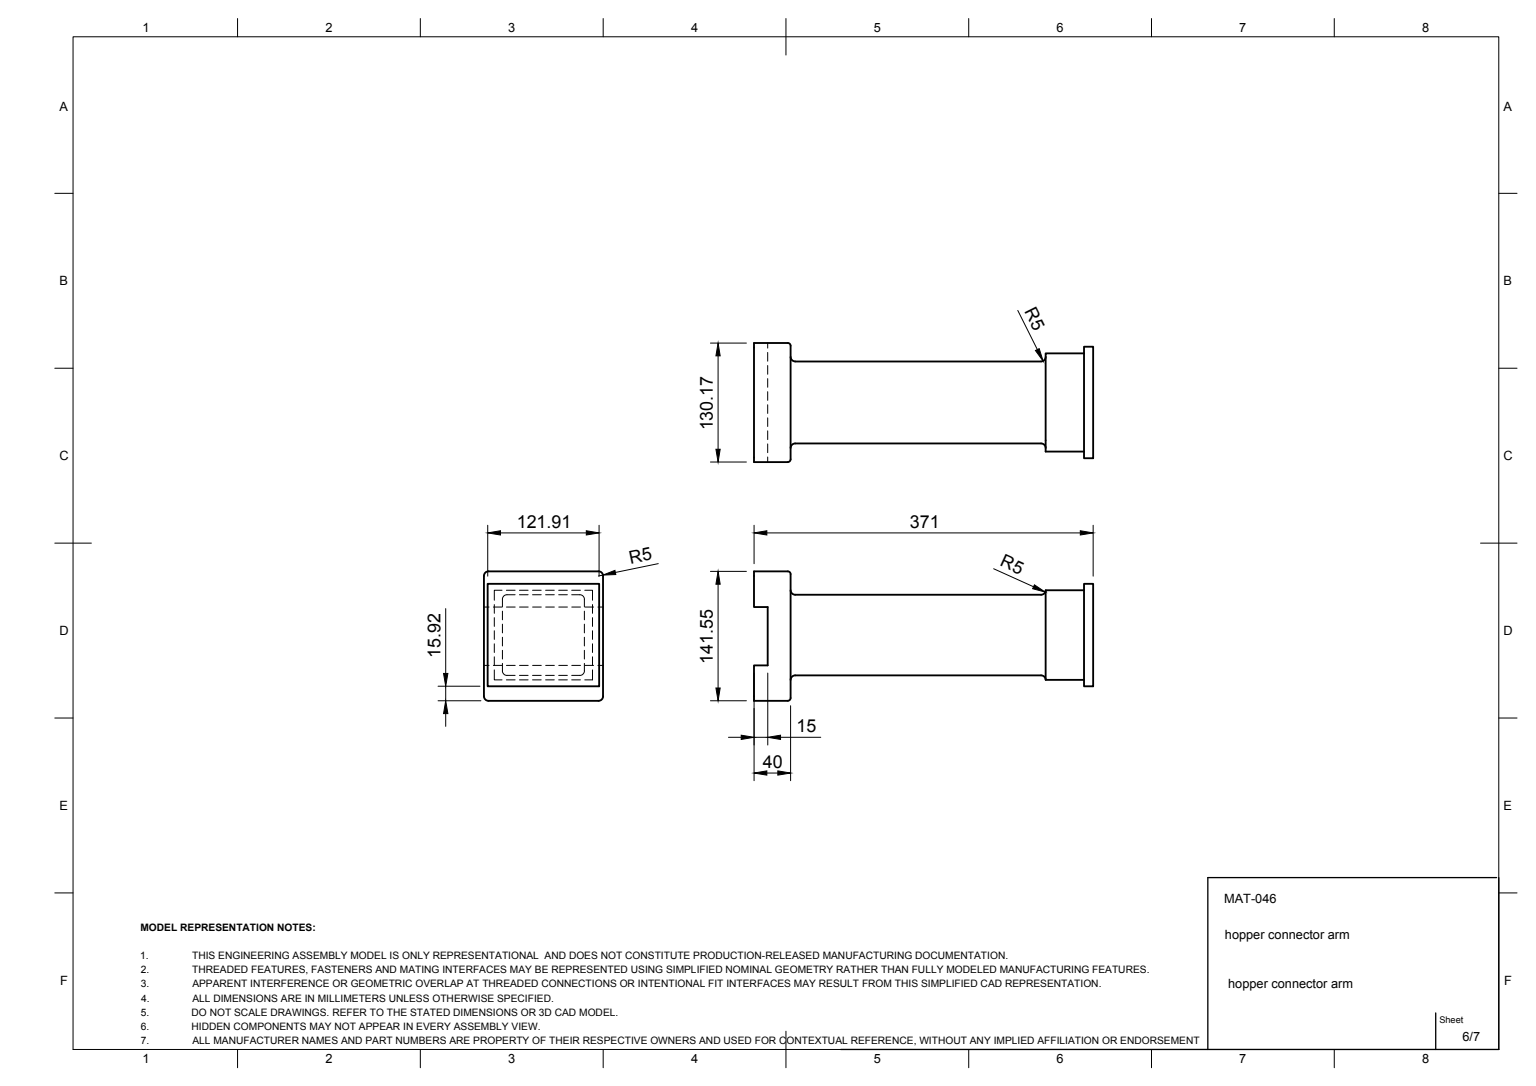
ISO-10303-21;
HEADER;
/* Generated by software containing ST-Developer
 * from STEP Tools, Inc. (www.steptools.com) 
 */

FILE_DESCRIPTION(
/* description */ ('STEP AP214'),
/* implementation_level */ '2;1');

FILE_NAME(
/* name */ 'hopper connector arm.step',
/* time_stamp */ '2026-11-14T22:16:48-08:00',
/* author */ (''),
/* organization */ (''),
/* preprocessor_version */ 'ST-DEVELOPER v20.2',
/* originating_system */ 'Autodesk Translation Framework v15.17.0.0',
/* authorisation */ '');

FILE_SCHEMA (('AUTOMOTIVE_DESIGN { 1 0 10303 214 3 1 1 }'));
ENDSEC;

DATA;
#10=MECHANICAL_DESIGN_GEOMETRIC_PRESENTATION_REPRESENTATION('',(#5499),#276462);
#4057=(
BOUNDED_SURFACE()
B_SPLINE_SURFACE(2,2,((#273891,#273892,#273893),(#273894,#273895,#273896),
(#273897,#273898,#273899)),.UNSPECIFIED.,.F.,.F.,.F.)
B_SPLINE_SURFACE_WITH_KNOTS((3,3),(3,3),(0.,1.57079632679491),(-3.14159265358979,
-1.5707963267949),.UNSPECIFIED.)
GEOMETRIC_REPRESENTATION_ITEM()
RATIONAL_B_SPLINE_SURFACE(((1.,0.707106781186548,1.),(0.707106781186546,
0.499999999999999,0.707106781186546),(1.,0.707106781186548,1.)))
REPRESENTATION_ITEM('')
SURFACE()
);
#4058=(
BOUNDED_SURFACE()
B_SPLINE_SURFACE(2,2,((#273906,#273907,#273908),(#273909,#273910,#273911),
(#273912,#273913,#273914)),.UNSPECIFIED.,.F.,.F.,.F.)
B_SPLINE_SURFACE_WITH_KNOTS((3,3),(3,3),(0.,1.57079632679491),(-1.5707963267949,
0.),.UNSPECIFIED.)
GEOMETRIC_REPRESENTATION_ITEM()
RATIONAL_B_SPLINE_SURFACE(((1.,0.707106781186547,1.),(0.707106781186542,
0.499999999999996,0.707106781186542),(1.,0.707106781186547,1.)))
REPRESENTATION_ITEM('')
SURFACE()
);
#4059=(
BOUNDED_SURFACE()
B_SPLINE_SURFACE(2,2,((#273916,#273917,#273918),(#273919,#273920,#273921),
(#273922,#273923,#273924)),.UNSPECIFIED.,.F.,.F.,.F.)
B_SPLINE_SURFACE_WITH_KNOTS((3,3),(3,3),(0.,1.57079632679491),(1.5707963267949,
3.14159265358979),.UNSPECIFIED.)
GEOMETRIC_REPRESENTATION_ITEM()
RATIONAL_B_SPLINE_SURFACE(((1.,0.707106781186548,1.),(0.707106781186542,
0.499999999999996,0.707106781186542),(1.,0.707106781186548,1.)))
REPRESENTATION_ITEM('')
SURFACE()
);
#4060=(
BOUNDED_SURFACE()
B_SPLINE_SURFACE(2,2,((#273930,#273931,#273932),(#273933,#273934,#273935),
(#273936,#273937,#273938)),.UNSPECIFIED.,.F.,.F.,.F.)
B_SPLINE_SURFACE_WITH_KNOTS((3,3),(3,3),(0.,1.57079632679491),(0.,1.5707963267949),
 .UNSPECIFIED.)
GEOMETRIC_REPRESENTATION_ITEM()
RATIONAL_B_SPLINE_SURFACE(((1.,0.707106781186548,1.),(0.707106781186542,
0.499999999999996,0.707106781186542),(1.,0.707106781186548,1.)))
REPRESENTATION_ITEM('')
SURFACE()
);
#4061=(
BOUNDED_SURFACE()
B_SPLINE_SURFACE(3,2,((#274053,#274054,#274055),(#274056,#274057,#274058),
(#274059,#274060,#274061),(#274062,#274063,#274064)),.UNSPECIFIED.,.F.,
 .F.,.F.)
B_SPLINE_SURFACE_WITH_KNOTS((4,4),(3,3),(0.00902295194197484,0.0107038053334674),
(0.,1.),.UNSPECIFIED.)
GEOMETRIC_REPRESENTATION_ITEM()
RATIONAL_B_SPLINE_SURFACE(((1.,0.717027218350901,1.),(1.,0.717027379451177,
1.),(1.,0.713716651700049,1.),(1.,0.707106781186548,1.)))
REPRESENTATION_ITEM('')
SURFACE()
);
#4062=(
BOUNDED_SURFACE()
B_SPLINE_SURFACE(3,2,((#274072,#274073,#274074),(#274075,#274076,#274077),
(#274078,#274079,#274080),(#274081,#274082,#274083)),.UNSPECIFIED.,.F.,
 .F.,.F.)
B_SPLINE_SURFACE_WITH_KNOTS((4,4),(3,3),(0.00902295194197483,0.0107038053334674),
(0.,1.),.UNSPECIFIED.)
GEOMETRIC_REPRESENTATION_ITEM()
RATIONAL_B_SPLINE_SURFACE(((1.,0.717027218350901,1.),(1.,0.717027379451176,
1.),(1.,0.713716651700055,1.),(1.,0.707106781186548,1.)))
REPRESENTATION_ITEM('')
SURFACE()
);
#4063=(
BOUNDED_SURFACE()
B_SPLINE_SURFACE(3,2,((#274085,#274086,#274087),(#274088,#274089,#274090),
(#274091,#274092,#274093),(#274094,#274095,#274096)),.UNSPECIFIED.,.F.,
 .F.,.F.)
B_SPLINE_SURFACE_WITH_KNOTS((4,4),(3,3),(0.00902295194197484,0.0107038053334674),
(0.,1.),.UNSPECIFIED.)
GEOMETRIC_REPRESENTATION_ITEM()
RATIONAL_B_SPLINE_SURFACE(((1.,0.717027218350901,1.),(1.,0.717027379451177,
1.),(1.,0.713716651700049,1.),(1.,0.707106781186548,1.)))
REPRESENTATION_ITEM('')
SURFACE()
);
#4064=(
BOUNDED_SURFACE()
B_SPLINE_SURFACE(3,2,((#274104,#274105,#274106),(#274107,#274108,#274109),
(#274110,#274111,#274112),(#274113,#274114,#274115)),.UNSPECIFIED.,.F.,
 .F.,.F.)
B_SPLINE_SURFACE_WITH_KNOTS((4,4),(3,3),(0.00902295194197484,0.0107038053334674),
(0.,1.),.UNSPECIFIED.)
GEOMETRIC_REPRESENTATION_ITEM()
RATIONAL_B_SPLINE_SURFACE(((1.,0.717027218350901,1.),(1.,0.717027379451177,
1.),(1.,0.713716651700049,1.),(1.,0.707106781186548,1.)))
REPRESENTATION_ITEM('')
SURFACE()
);
#5456=B_SPLINE_CURVE_WITH_KNOTS('',3,(#273943,#273944,#273945,#273946,#273947,
#273948,#273949,#273950,#273951,#273952),.UNSPECIFIED.,.F.,.F.,(4,3,3,4),
(0.,0.000338853006806234,0.000677883858435526,0.00084344531229996),
 .UNSPECIFIED.);
#5457=B_SPLINE_CURVE_WITH_KNOTS('',3,(#273956,#273957,#273958,#273959,#273960,
#273961,#273962,#273963,#273964,#273965),.UNSPECIFIED.,.F.,.F.,(4,3,3,4),
(0.,0.000336488810998176,0.000673156284667907,0.000840479374202616),
 .UNSPECIFIED.);
#5458=B_SPLINE_CURVE_WITH_KNOTS('',3,(#273970,#273971,#273972,#273973,#273974,
#273975,#273976,#273977,#273978,#273979),.UNSPECIFIED.,.F.,.F.,(4,3,3,4),
(0.,0.000336488811000739,0.000673156284671631,0.000840479374202609),
 .UNSPECIFIED.);
#5459=B_SPLINE_CURVE_WITH_KNOTS('',3,(#273985,#273986,#273987,#273988,#273989,
#273990,#273991,#273992,#273993,#273994),.UNSPECIFIED.,.F.,.F.,(4,3,3,4),
(0.,0.000338853006809123,0.000677883858442031,0.000843445312299953),
 .UNSPECIFIED.);
#5464=SHAPE_REPRESENTATION_RELATIONSHIP('SRR','None',#276492,#5470);
#5470=ADVANCED_BREP_SHAPE_REPRESENTATION('',(#5528),#276460);
#5499=STYLED_ITEM('',(#276527),#5528);
#5528=MANIFOLD_SOLID_BREP('Body1',#98724);
#6314=TOROIDAL_SURFACE('',#110940,10.,5.);
#6315=TOROIDAL_SURFACE('',#110947,10.,5.);
#6316=TOROIDAL_SURFACE('',#110949,10.,5.);
#6317=TOROIDAL_SURFACE('',#110955,10.,5.);
#6318=TOROIDAL_SURFACE('',#110956,10.,5.);
#6319=TOROIDAL_SURFACE('',#110964,10.,5.);
#6320=TOROIDAL_SURFACE('',#110968,10.,5.);
#6321=TOROIDAL_SURFACE('',#110975,10.,5.);
#6442=FACE_BOUND('',#19499,.T.);
#6443=FACE_BOUND('',#19546,.T.);
#7328=PLANE('',#110876);
#7329=PLANE('',#110877);
#7330=PLANE('',#110880);
#7331=PLANE('',#110881);
#7332=PLANE('',#110882);
#7333=PLANE('',#110883);
#7334=PLANE('',#110884);
#7335=PLANE('',#110893);
#7336=PLANE('',#110894);
#7337=PLANE('',#110895);
#7338=PLANE('',#110896);
#7339=PLANE('',#110933);
#7340=PLANE('',#110934);
#7341=PLANE('',#110935);
#7342=PLANE('',#110936);
#7343=PLANE('',#110937);
#7344=PLANE('',#110976);
#7345=PLANE('',#110977);
#7346=PLANE('',#110978);
#7347=PLANE('',#110979);
#7348=PLANE('',#110980);
#7349=PLANE('',#110981);
#7350=PLANE('',#110982);
#7351=PLANE('',#110983);
#7352=PLANE('',#110984);
#7353=PLANE('',#110985);
#13262=FACE_OUTER_BOUND('',#19492,.T.);
#13263=FACE_OUTER_BOUND('',#19493,.T.);
#13264=FACE_OUTER_BOUND('',#19494,.T.);
#13265=FACE_OUTER_BOUND('',#19495,.T.);
#13266=FACE_OUTER_BOUND('',#19496,.T.);
#13267=FACE_OUTER_BOUND('',#19497,.T.);
#13268=FACE_OUTER_BOUND('',#19498,.T.);
#13269=FACE_OUTER_BOUND('',#19500,.T.);
#13270=FACE_OUTER_BOUND('',#19501,.T.);
#13271=FACE_OUTER_BOUND('',#19502,.T.);
#13272=FACE_OUTER_BOUND('',#19503,.T.);
#13273=FACE_OUTER_BOUND('',#19504,.T.);
#13274=FACE_OUTER_BOUND('',#19505,.T.);
#13275=FACE_OUTER_BOUND('',#19506,.T.);
#13276=FACE_OUTER_BOUND('',#19507,.T.);
#13277=FACE_OUTER_BOUND('',#19508,.T.);
#13278=FACE_OUTER_BOUND('',#19509,.T.);
#13279=FACE_OUTER_BOUND('',#19510,.T.);
#13280=FACE_OUTER_BOUND('',#19511,.T.);
#13281=FACE_OUTER_BOUND('',#19512,.T.);
#13282=FACE_OUTER_BOUND('',#19513,.T.);
#13283=FACE_OUTER_BOUND('',#19514,.T.);
#13284=FACE_OUTER_BOUND('',#19515,.T.);
#13285=FACE_OUTER_BOUND('',#19516,.T.);
#13286=FACE_OUTER_BOUND('',#19517,.T.);
#13287=FACE_OUTER_BOUND('',#19518,.T.);
#13288=FACE_OUTER_BOUND('',#19519,.T.);
#13289=FACE_OUTER_BOUND('',#19520,.T.);
#13290=FACE_OUTER_BOUND('',#19521,.T.);
#13291=FACE_OUTER_BOUND('',#19522,.T.);
#13292=FACE_OUTER_BOUND('',#19523,.T.);
#13293=FACE_OUTER_BOUND('',#19524,.T.);
#13294=FACE_OUTER_BOUND('',#19525,.T.);
#13295=FACE_OUTER_BOUND('',#19526,.T.);
#13296=FACE_OUTER_BOUND('',#19527,.T.);
#13297=FACE_OUTER_BOUND('',#19528,.T.);
#13298=FACE_OUTER_BOUND('',#19529,.T.);
#13299=FACE_OUTER_BOUND('',#19530,.T.);
#13300=FACE_OUTER_BOUND('',#19531,.T.);
#13301=FACE_OUTER_BOUND('',#19532,.T.);
#13302=FACE_OUTER_BOUND('',#19533,.T.);
#13303=FACE_OUTER_BOUND('',#19534,.T.);
#13304=FACE_OUTER_BOUND('',#19535,.T.);
#13305=FACE_OUTER_BOUND('',#19536,.T.);
#13306=FACE_OUTER_BOUND('',#19537,.T.);
#13307=FACE_OUTER_BOUND('',#19538,.T.);
#13308=FACE_OUTER_BOUND('',#19539,.T.);
#13309=FACE_OUTER_BOUND('',#19540,.T.);
#13310=FACE_OUTER_BOUND('',#19541,.T.);
#13311=FACE_OUTER_BOUND('',#19542,.T.);
#13312=FACE_OUTER_BOUND('',#19543,.T.);
#13313=FACE_OUTER_BOUND('',#19544,.T.);
#13314=FACE_OUTER_BOUND('',#19545,.T.);
#13315=FACE_OUTER_BOUND('',#19547,.T.);
#13316=FACE_OUTER_BOUND('',#19548,.T.);
#13317=FACE_OUTER_BOUND('',#19549,.T.);
#13318=FACE_OUTER_BOUND('',#19550,.T.);
#13319=FACE_OUTER_BOUND('',#19551,.T.);
#13320=FACE_OUTER_BOUND('',#19552,.T.);
#13321=FACE_OUTER_BOUND('',#19553,.T.);
#13322=FACE_OUTER_BOUND('',#19554,.T.);
#13323=FACE_OUTER_BOUND('',#19555,.T.);
#19492=EDGE_LOOP('',(#87733,#87734,#87735,#87736));
#19493=EDGE_LOOP('',(#87737,#87738,#87739,#87740,#87741,#87742));
#19494=EDGE_LOOP('',(#87743,#87744,#87745,#87746,#87747,#87748,#87749,#87750));
#19495=EDGE_LOOP('',(#87751,#87752,#87753,#87754));
#19496=EDGE_LOOP('',(#87755,#87756,#87757,#87758,#87759,#87760,#87761,#87762));
#19497=EDGE_LOOP('',(#87763,#87764,#87765,#87766));
#19498=EDGE_LOOP('',(#87767,#87768,#87769,#87770,#87771,#87772,#87773,#87774));
#19499=EDGE_LOOP('',(#87775,#87776,#87777,#87778,#87779,#87780,#87781,#87782));
#19500=EDGE_LOOP('',(#87783,#87784,#87785,#87786));
#19501=EDGE_LOOP('',(#87787,#87788,#87789,#87790));
#19502=EDGE_LOOP('',(#87791,#87792,#87793,#87794));
#19503=EDGE_LOOP('',(#87795,#87796,#87797,#87798));
#19504=EDGE_LOOP('',(#87799,#87800,#87801,#87802));
#19505=EDGE_LOOP('',(#87803,#87804,#87805,#87806));
#19506=EDGE_LOOP('',(#87807,#87808,#87809,#87810));
#19507=EDGE_LOOP('',(#87811,#87812,#87813,#87814));
#19508=EDGE_LOOP('',(#87815,#87816,#87817,#87818));
#19509=EDGE_LOOP('',(#87819,#87820,#87821,#87822));
#19510=EDGE_LOOP('',(#87823,#87824,#87825,#87826));
#19511=EDGE_LOOP('',(#87827,#87828,#87829,#87830));
#19512=EDGE_LOOP('',(#87831,#87832,#87833,#87834));
#19513=EDGE_LOOP('',(#87835,#87836,#87837,#87838));
#19514=EDGE_LOOP('',(#87839,#87840,#87841,#87842));
#19515=EDGE_LOOP('',(#87843,#87844,#87845,#87846));
#19516=EDGE_LOOP('',(#87847,#87848,#87849,#87850,#87851));
#19517=EDGE_LOOP('',(#87852,#87853,#87854,#87855,#87856));
#19518=EDGE_LOOP('',(#87857,#87858,#87859,#87860,#87861));
#19519=EDGE_LOOP('',(#87862,#87863,#87864,#87865,#87866));
#19520=EDGE_LOOP('',(#87867,#87868,#87869,#87870));
#19521=EDGE_LOOP('',(#87871,#87872,#87873,#87874,#87875,#87876,#87877,#87878));
#19522=EDGE_LOOP('',(#87879,#87880,#87881,#87882));
#19523=EDGE_LOOP('',(#87883,#87884,#87885,#87886,#87887,#87888,#87889,#87890));
#19524=EDGE_LOOP('',(#87891,#87892,#87893,#87894,#87895,#87896));
#19525=EDGE_LOOP('',(#87897,#87898,#87899,#87900));
#19526=EDGE_LOOP('',(#87901,#87902,#87903,#87904));
#19527=EDGE_LOOP('',(#87905,#87906,#87907,#87908));
#19528=EDGE_LOOP('',(#87909,#87910,#87911,#87912));
#19529=EDGE_LOOP('',(#87913,#87914,#87915,#87916));
#19530=EDGE_LOOP('',(#87917,#87918,#87919,#87920));
#19531=EDGE_LOOP('',(#87921,#87922,#87923,#87924));
#19532=EDGE_LOOP('',(#87925,#87926,#87927,#87928));
#19533=EDGE_LOOP('',(#87929,#87930,#87931,#87932));
#19534=EDGE_LOOP('',(#87933,#87934,#87935,#87936));
#19535=EDGE_LOOP('',(#87937,#87938,#87939,#87940));
#19536=EDGE_LOOP('',(#87941,#87942,#87943,#87944));
#19537=EDGE_LOOP('',(#87945,#87946,#87947,#87948));
#19538=EDGE_LOOP('',(#87949,#87950,#87951,#87952));
#19539=EDGE_LOOP('',(#87953,#87954,#87955,#87956));
#19540=EDGE_LOOP('',(#87957,#87958,#87959,#87960));
#19541=EDGE_LOOP('',(#87961,#87962,#87963,#87964));
#19542=EDGE_LOOP('',(#87965,#87966,#87967,#87968));
#19543=EDGE_LOOP('',(#87969,#87970,#87971,#87972));
#19544=EDGE_LOOP('',(#87973,#87974,#87975,#87976));
#19545=EDGE_LOOP('',(#87977,#87978,#87979,#87980));
#19546=EDGE_LOOP('',(#87981,#87982,#87983,#87984));
#19547=EDGE_LOOP('',(#87985,#87986,#87987,#87988));
#19548=EDGE_LOOP('',(#87989,#87990,#87991,#87992));
#19549=EDGE_LOOP('',(#87993,#87994,#87995,#87996));
#19550=EDGE_LOOP('',(#87997,#87998,#87999,#88000));
#19551=EDGE_LOOP('',(#88001,#88002,#88003,#88004));
#19552=EDGE_LOOP('',(#88005,#88006,#88007,#88008));
#19553=EDGE_LOOP('',(#88009,#88010,#88011,#88012,#88013,#88014));
#19554=EDGE_LOOP('',(#88015,#88016,#88017,#88018));
#19555=EDGE_LOOP('',(#88019,#88020,#88021,#88022,#88023,#88024));
#24245=LINE('',#273745,#29472);
#24246=LINE('',#273747,#29473);
#24247=LINE('',#273749,#29474);
#24248=LINE('',#273750,#29475);
#24249=LINE('',#273754,#29476);
#24250=LINE('',#273758,#29477);
#24251=LINE('',#273760,#29478);
#24252=LINE('',#273762,#29479);
#24253=LINE('',#273767,#29480);
#24254=LINE('',#273769,#29481);
#24255=LINE('',#273771,#29482);
#24256=LINE('',#273773,#29483);
#24257=LINE('',#273774,#29484);
#24258=LINE('',#273776,#29485);
#24259=LINE('',#273777,#29486);
#24260=LINE('',#273781,#29487);
#24261=LINE('',#273783,#29488);
#24262=LINE('',#273785,#29489);
#24263=LINE('',#273786,#29490);
#24264=LINE('',#273790,#29491);
#24265=LINE('',#273792,#29492);
#24266=LINE('',#273794,#29493);
#24267=LINE('',#273796,#29494);
#24268=LINE('',#273797,#29495);
#24269=LINE('',#273799,#29496);
#24270=LINE('',#273800,#29497);
#24271=LINE('',#273804,#29498);
#24272=LINE('',#273806,#29499);
#24273=LINE('',#273808,#29500);
#24274=LINE('',#273809,#29501);
#24275=LINE('',#273813,#29502);
#24276=LINE('',#273817,#29503);
#24277=LINE('',#273821,#29504);
#24278=LINE('',#273825,#29505);
#24279=LINE('',#273829,#29506);
#24280=LINE('',#273833,#29507);
#24281=LINE('',#273837,#29508);
#24282=LINE('',#273841,#29509);
#24283=LINE('',#273846,#29510);
#24284=LINE('',#273848,#29511);
#24285=LINE('',#273850,#29512);
#24286=LINE('',#273851,#29513);
#24287=LINE('',#273855,#29514);
#24288=LINE('',#273857,#29515);
#24289=LINE('',#273859,#29516);
#24290=LINE('',#273860,#29517);
#24291=LINE('',#273864,#29518);
#24292=LINE('',#273866,#29519);
#24293=LINE('',#273868,#29520);
#24294=LINE('',#273869,#29521);
#24295=LINE('',#273873,#29522);
#24296=LINE('',#273875,#29523);
#24297=LINE('',#273877,#29524);
#24298=LINE('',#273878,#29525);
#24299=LINE('',#273997,#29526);
#24300=LINE('',#273999,#29527);
#24301=LINE('',#274000,#29528);
#24302=LINE('',#274003,#29529);
#24303=LINE('',#274005,#29530);
#24304=LINE('',#274007,#29531);
#24305=LINE('',#274009,#29532);
#24306=LINE('',#274011,#29533);
#24307=LINE('',#274012,#29534);
#24308=LINE('',#274015,#29535);
#24309=LINE('',#274017,#29536);
#24310=LINE('',#274018,#29537);
#24311=LINE('',#274021,#29538);
#24312=LINE('',#274023,#29539);
#24313=LINE('',#274025,#29540);
#24314=LINE('',#274026,#29541);
#24315=LINE('',#274027,#29542);
#24316=LINE('',#274031,#29543);
#24317=LINE('',#274121,#29544);
#24318=LINE('',#274123,#29545);
#24319=LINE('',#274125,#29546);
#24320=LINE('',#274126,#29547);
#24321=LINE('',#274129,#29548);
#24322=LINE('',#274131,#29549);
#24323=LINE('',#274132,#29550);
#24324=LINE('',#274135,#29551);
#24325=LINE('',#274136,#29552);
#24326=LINE('',#274139,#29553);
#24327=LINE('',#274140,#29554);
#24328=LINE('',#274142,#29555);
#24329=LINE('',#274145,#29556);
#24330=LINE('',#274148,#29557);
#29472=VECTOR('',#140110,1000.);
#29473=VECTOR('',#140111,1000.);
#29474=VECTOR('',#140112,1000.);
#29475=VECTOR('',#140113,1000.);
#29476=VECTOR('',#140116,1000.);
#29477=VECTOR('',#140119,1000.);
#29478=VECTOR('',#140120,1000.);
#29479=VECTOR('',#140121,1000.);
#29480=VECTOR('',#140126,1000.);
#29481=VECTOR('',#140127,1000.);
#29482=VECTOR('',#140128,1000.);
#29483=VECTOR('',#140129,1000.);
#29484=VECTOR('',#140130,1000.);
#29485=VECTOR('',#140131,1000.);
#29486=VECTOR('',#140132,1000.);
#29487=VECTOR('',#140135,1000.);
#29488=VECTOR('',#140136,1000.);
#29489=VECTOR('',#140137,1000.);
#29490=VECTOR('',#140138,1000.);
#29491=VECTOR('',#140141,1000.);
#29492=VECTOR('',#140142,1000.);
#29493=VECTOR('',#140143,1000.);
#29494=VECTOR('',#140144,1000.);
#29495=VECTOR('',#140145,1000.);
#29496=VECTOR('',#140146,1000.);
#29497=VECTOR('',#140147,1000.);
#29498=VECTOR('',#140150,1000.);
#29499=VECTOR('',#140151,1000.);
#29500=VECTOR('',#140152,1000.);
#29501=VECTOR('',#140153,1000.);
#29502=VECTOR('',#140156,1000.);
#29503=VECTOR('',#140159,1000.);
#29504=VECTOR('',#140162,1000.);
#29505=VECTOR('',#140165,1000.);
#29506=VECTOR('',#140168,1000.);
#29507=VECTOR('',#140171,1000.);
#29508=VECTOR('',#140174,1000.);
#29509=VECTOR('',#140177,1000.);
#29510=VECTOR('',#140182,1000.);
#29511=VECTOR('',#140183,1000.);
#29512=VECTOR('',#140184,1000.);
#29513=VECTOR('',#140185,1000.);
#29514=VECTOR('',#140188,1000.);
#29515=VECTOR('',#140189,1000.);
#29516=VECTOR('',#140190,1000.);
#29517=VECTOR('',#140191,1000.);
#29518=VECTOR('',#140194,1000.);
#29519=VECTOR('',#140195,1000.);
#29520=VECTOR('',#140196,1000.);
#29521=VECTOR('',#140197,1000.);
#29522=VECTOR('',#140200,1000.);
#29523=VECTOR('',#140201,1000.);
#29524=VECTOR('',#140202,1000.);
#29525=VECTOR('',#140203,1000.);
#29526=VECTOR('',#140278,1000.);
#29527=VECTOR('',#140279,1000.);
#29528=VECTOR('',#140280,1000.);
#29529=VECTOR('',#140283,1000.);
#29530=VECTOR('',#140284,1000.);
#29531=VECTOR('',#140285,1000.);
#29532=VECTOR('',#140286,1000.);
#29533=VECTOR('',#140287,1000.);
#29534=VECTOR('',#140288,1000.);
#29535=VECTOR('',#140291,1000.);
#29536=VECTOR('',#140292,1000.);
#29537=VECTOR('',#140293,1000.);
#29538=VECTOR('',#140296,1000.);
#29539=VECTOR('',#140297,1000.);
#29540=VECTOR('',#140298,1000.);
#29541=VECTOR('',#140299,1000.);
#29542=VECTOR('',#140300,1000.);
#29543=VECTOR('',#140303,1000.);
#29544=VECTOR('',#140382,1000.);
#29545=VECTOR('',#140383,1000.);
#29546=VECTOR('',#140384,1000.);
#29547=VECTOR('',#140385,1000.);
#29548=VECTOR('',#140388,1000.);
#29549=VECTOR('',#140389,1000.);
#29550=VECTOR('',#140390,1000.);
#29551=VECTOR('',#140393,1000.);
#29552=VECTOR('',#140394,1000.);
#29553=VECTOR('',#140397,1000.);
#29554=VECTOR('',#140398,1000.);
#29555=VECTOR('',#140401,1000.);
#29556=VECTOR('',#140406,1000.);
#29557=VECTOR('',#140411,1000.);
#36223=CIRCLE('',#110878,10.);
#36224=CIRCLE('',#110879,10.);
#36225=CIRCLE('',#110885,2.);
#36226=CIRCLE('',#110886,2.);
#36227=CIRCLE('',#110887,2.);
#36228=CIRCLE('',#110888,2.);
#36229=CIRCLE('',#110889,10.);
#36230=CIRCLE('',#110890,10.);
#36231=CIRCLE('',#110891,10.);
#36232=CIRCLE('',#110892,10.);
#36233=CIRCLE('',#110898,5.);
#36234=CIRCLE('',#110899,5.);
#36235=CIRCLE('',#110901,5.);
#36236=CIRCLE('',#110902,5.);
#36237=CIRCLE('',#110904,5.);
#36238=CIRCLE('',#110905,5.);
#36239=CIRCLE('',#110907,5.);
#36240=CIRCLE('',#110908,5.);
#36241=CIRCLE('',#110909,3.);
#36242=CIRCLE('',#110910,3.);
#36243=CIRCLE('',#110912,3.);
#36244=CIRCLE('',#110914,3.);
#36245=CIRCLE('',#110915,3.);
#36246=CIRCLE('',#110916,3.);
#36247=CIRCLE('',#110918,3.);
#36248=CIRCLE('',#110920,3.);
#36249=CIRCLE('',#110922,5.);
#36250=CIRCLE('',#110923,5.);
#36251=CIRCLE('',#110925,5.);
#36252=CIRCLE('',#110926,5.);
#36253=CIRCLE('',#110928,5.);
#36254=CIRCLE('',#110929,5.);
#36255=CIRCLE('',#110931,5.);
#36256=CIRCLE('',#110932,5.);
#36257=CIRCLE('',#110938,10.);
#36258=CIRCLE('',#110939,10.);
#36259=CIRCLE('',#110941,5.);
#36260=CIRCLE('',#110942,5.);
#36261=CIRCLE('',#110944,5.);
#36262=CIRCLE('',#110946,5.);
#36263=CIRCLE('',#110948,5.);
#36264=CIRCLE('',#110950,5.);
#36265=CIRCLE('',#110952,5.);
#36266=CIRCLE('',#110954,5.);
#36267=CIRCLE('',#110957,5.);
#36268=CIRCLE('',#110958,5.);
#36269=CIRCLE('',#110959,5.);
#36270=CIRCLE('',#110961,5.);
#36271=CIRCLE('',#110963,5.);
#36272=CIRCLE('',#110965,5.);
#36273=CIRCLE('',#110966,5.);
#36274=CIRCLE('',#110967,5.);
#36275=CIRCLE('',#110969,5.);
#36276=CIRCLE('',#110971,5.);
#36277=CIRCLE('',#110973,5.);
#36278=CIRCLE('',#110974,5.);
#44647=VERTEX_POINT('',#273743);
#44648=VERTEX_POINT('',#273744);
#44649=VERTEX_POINT('',#273746);
#44650=VERTEX_POINT('',#273748);
#44651=VERTEX_POINT('',#273752);
#44652=VERTEX_POINT('',#273753);
#44653=VERTEX_POINT('',#273755);
#44654=VERTEX_POINT('',#273757);
#44655=VERTEX_POINT('',#273759);
#44656=VERTEX_POINT('',#273761);
#44657=VERTEX_POINT('',#273765);
#44658=VERTEX_POINT('',#273766);
#44659=VERTEX_POINT('',#273768);
#44660=VERTEX_POINT('',#273770);
#44661=VERTEX_POINT('',#273772);
#44662=VERTEX_POINT('',#273775);
#44663=VERTEX_POINT('',#273779);
#44664=VERTEX_POINT('',#273780);
#44665=VERTEX_POINT('',#273782);
#44666=VERTEX_POINT('',#273784);
#44667=VERTEX_POINT('',#273788);
#44668=VERTEX_POINT('',#273789);
#44669=VERTEX_POINT('',#273791);
#44670=VERTEX_POINT('',#273793);
#44671=VERTEX_POINT('',#273795);
#44672=VERTEX_POINT('',#273798);
#44673=VERTEX_POINT('',#273802);
#44674=VERTEX_POINT('',#273803);
#44675=VERTEX_POINT('',#273805);
#44676=VERTEX_POINT('',#273807);
#44677=VERTEX_POINT('',#273811);
#44678=VERTEX_POINT('',#273812);
#44679=VERTEX_POINT('',#273814);
#44680=VERTEX_POINT('',#273816);
#44681=VERTEX_POINT('',#273818);
#44682=VERTEX_POINT('',#273820);
#44683=VERTEX_POINT('',#273822);
#44684=VERTEX_POINT('',#273824);
#44685=VERTEX_POINT('',#273827);
#44686=VERTEX_POINT('',#273828);
#44687=VERTEX_POINT('',#273830);
#44688=VERTEX_POINT('',#273832);
#44689=VERTEX_POINT('',#273834);
#44690=VERTEX_POINT('',#273836);
#44691=VERTEX_POINT('',#273838);
#44692=VERTEX_POINT('',#273840);
#44693=VERTEX_POINT('',#273844);
#44694=VERTEX_POINT('',#273845);
#44695=VERTEX_POINT('',#273847);
#44696=VERTEX_POINT('',#273849);
#44697=VERTEX_POINT('',#273853);
#44698=VERTEX_POINT('',#273854);
#44699=VERTEX_POINT('',#273856);
#44700=VERTEX_POINT('',#273858);
#44701=VERTEX_POINT('',#273862);
#44702=VERTEX_POINT('',#273863);
#44703=VERTEX_POINT('',#273865);
#44704=VERTEX_POINT('',#273867);
#44705=VERTEX_POINT('',#273871);
#44706=VERTEX_POINT('',#273872);
#44707=VERTEX_POINT('',#273874);
#44708=VERTEX_POINT('',#273876);
#44709=VERTEX_POINT('',#273941);
#44710=VERTEX_POINT('',#273955);
#44711=VERTEX_POINT('',#273969);
#44712=VERTEX_POINT('',#273983);
#44713=VERTEX_POINT('',#273996);
#44714=VERTEX_POINT('',#273998);
#44715=VERTEX_POINT('',#274002);
#44716=VERTEX_POINT('',#274004);
#44717=VERTEX_POINT('',#274006);
#44718=VERTEX_POINT('',#274008);
#44719=VERTEX_POINT('',#274010);
#44720=VERTEX_POINT('',#274014);
#44721=VERTEX_POINT('',#274016);
#44722=VERTEX_POINT('',#274020);
#44723=VERTEX_POINT('',#274022);
#44724=VERTEX_POINT('',#274024);
#44725=VERTEX_POINT('',#274029);
#44726=VERTEX_POINT('',#274030);
#44727=VERTEX_POINT('',#274119);
#44728=VERTEX_POINT('',#274120);
#44729=VERTEX_POINT('',#274122);
#44730=VERTEX_POINT('',#274124);
#44731=VERTEX_POINT('',#274128);
#44732=VERTEX_POINT('',#274130);
#44733=VERTEX_POINT('',#274134);
#44734=VERTEX_POINT('',#274138);
#59145=EDGE_CURVE('',#44647,#44648,#24245,.T.);
#59146=EDGE_CURVE('',#44649,#44647,#24246,.T.);
#59147=EDGE_CURVE('',#44650,#44649,#24247,.T.);
#59148=EDGE_CURVE('',#44648,#44650,#24248,.T.);
#59149=EDGE_CURVE('',#44651,#44652,#24249,.T.);
#59150=EDGE_CURVE('',#44652,#44653,#36223,.T.);
#59151=EDGE_CURVE('',#44654,#44653,#24250,.T.);
#59152=EDGE_CURVE('',#44655,#44654,#24251,.T.);
#59153=EDGE_CURVE('',#44656,#44655,#24252,.T.);
#59154=EDGE_CURVE('',#44656,#44651,#36224,.T.);
#59155=EDGE_CURVE('',#44657,#44658,#24253,.T.);
#59156=EDGE_CURVE('',#44658,#44659,#24254,.T.);
#59157=EDGE_CURVE('',#44659,#44660,#24255,.T.);
#59158=EDGE_CURVE('',#44661,#44660,#24256,.T.);
#59159=EDGE_CURVE('',#44661,#44649,#24257,.T.);
#59160=EDGE_CURVE('',#44662,#44647,#24258,.T.);
#59161=EDGE_CURVE('',#44657,#44662,#24259,.T.);
#59162=EDGE_CURVE('',#44663,#44664,#24260,.T.);
#59163=EDGE_CURVE('',#44664,#44665,#24261,.T.);
#59164=EDGE_CURVE('',#44665,#44666,#24262,.T.);
#59165=EDGE_CURVE('',#44663,#44666,#24263,.T.);
#59166=EDGE_CURVE('',#44667,#44668,#24264,.T.);
#59167=EDGE_CURVE('',#44668,#44669,#24265,.T.);
#59168=EDGE_CURVE('',#44669,#44670,#24266,.T.);
#59169=EDGE_CURVE('',#44671,#44670,#24267,.T.);
#59170=EDGE_CURVE('',#44671,#44648,#24268,.T.);
#59171=EDGE_CURVE('',#44672,#44650,#24269,.T.);
#59172=EDGE_CURVE('',#44667,#44672,#24270,.T.);
#59173=EDGE_CURVE('',#44673,#44674,#24271,.T.);
#59174=EDGE_CURVE('',#44674,#44675,#24272,.T.);
#59175=EDGE_CURVE('',#44675,#44676,#24273,.T.);
#59176=EDGE_CURVE('',#44673,#44676,#24274,.T.);
#59177=EDGE_CURVE('',#44677,#44678,#24275,.T.);
#59178=EDGE_CURVE('',#44678,#44679,#36225,.T.);
#59179=EDGE_CURVE('',#44679,#44680,#24276,.T.);
#59180=EDGE_CURVE('',#44680,#44681,#36226,.T.);
#59181=EDGE_CURVE('',#44681,#44682,#24277,.T.);
#59182=EDGE_CURVE('',#44682,#44683,#36227,.T.);
#59183=EDGE_CURVE('',#44683,#44684,#24278,.T.);
#59184=EDGE_CURVE('',#44684,#44677,#36228,.T.);
#59185=EDGE_CURVE('',#44685,#44686,#24279,.T.);
#59186=EDGE_CURVE('',#44686,#44687,#36229,.T.);
#59187=EDGE_CURVE('',#44687,#44688,#24280,.T.);
#59188=EDGE_CURVE('',#44688,#44689,#36230,.T.);
#59189=EDGE_CURVE('',#44689,#44690,#24281,.T.);
#59190=EDGE_CURVE('',#44690,#44691,#36231,.T.);
#59191=EDGE_CURVE('',#44691,#44692,#24282,.T.);
#59192=EDGE_CURVE('',#44692,#44685,#36232,.T.);
#59193=EDGE_CURVE('',#44693,#44694,#24283,.T.);
#59194=EDGE_CURVE('',#44694,#44695,#24284,.T.);
#59195=EDGE_CURVE('',#44695,#44696,#24285,.T.);
#59196=EDGE_CURVE('',#44696,#44693,#24286,.T.);
#59197=EDGE_CURVE('',#44697,#44698,#24287,.T.);
#59198=EDGE_CURVE('',#44698,#44699,#24288,.T.);
#59199=EDGE_CURVE('',#44699,#44700,#24289,.T.);
#59200=EDGE_CURVE('',#44700,#44697,#24290,.T.);
#59201=EDGE_CURVE('',#44701,#44702,#24291,.T.);
#59202=EDGE_CURVE('',#44702,#44703,#24292,.T.);
#59203=EDGE_CURVE('',#44703,#44704,#24293,.T.);
#59204=EDGE_CURVE('',#44704,#44701,#24294,.T.);
#59205=EDGE_CURVE('',#44705,#44706,#24295,.T.);
#59206=EDGE_CURVE('',#44706,#44707,#24296,.T.);
#59207=EDGE_CURVE('',#44707,#44708,#24297,.T.);
#59208=EDGE_CURVE('',#44708,#44705,#24298,.T.);
#59209=EDGE_CURVE('',#44659,#44674,#36233,.T.);
#59210=EDGE_CURVE('',#44660,#44673,#36234,.T.);
#59211=EDGE_CURVE('',#44669,#44664,#36235,.T.);
#59212=EDGE_CURVE('',#44670,#44663,#36236,.T.);
#59213=EDGE_CURVE('',#44665,#44658,#36237,.T.);
#59214=EDGE_CURVE('',#44666,#44657,#36238,.T.);
#59215=EDGE_CURVE('',#44675,#44668,#36239,.T.);
#59216=EDGE_CURVE('',#44676,#44667,#36240,.T.);
#59217=EDGE_CURVE('',#44658,#44682,#36241,.T.);
#59218=EDGE_CURVE('',#44683,#44665,#36242,.T.);
#59219=EDGE_CURVE('',#44684,#44664,#36243,.T.);
#59220=EDGE_CURVE('',#44659,#44681,#36244,.T.);
#59221=EDGE_CURVE('',#44677,#44669,#36245,.T.);
#59222=EDGE_CURVE('',#44674,#44680,#36246,.T.);
#59223=EDGE_CURVE('',#44678,#44668,#36247,.T.);
#59224=EDGE_CURVE('',#44675,#44679,#36248,.T.);
#59225=EDGE_CURVE('',#44707,#44694,#36249,.T.);
#59226=EDGE_CURVE('',#44693,#44709,#36250,.T.);
#59227=EDGE_CURVE('',#44709,#44708,#5456,.T.);
#59228=EDGE_CURVE('',#44703,#44706,#36251,.T.);
#59229=EDGE_CURVE('',#44705,#44710,#5457,.T.);
#59230=EDGE_CURVE('',#44710,#44704,#36252,.T.);
#59231=EDGE_CURVE('',#44695,#44700,#36253,.T.);
#59232=EDGE_CURVE('',#44699,#44711,#5458,.T.);
#59233=EDGE_CURVE('',#44711,#44696,#36254,.T.);
#59234=EDGE_CURVE('',#44697,#44702,#36255,.T.);
#59235=EDGE_CURVE('',#44701,#44712,#36256,.T.);
#59236=EDGE_CURVE('',#44712,#44698,#5459,.T.);
#59237=EDGE_CURVE('',#44713,#44654,#24299,.T.);
#59238=EDGE_CURVE('',#44714,#44713,#24300,.T.);
#59239=EDGE_CURVE('',#44714,#44655,#24301,.T.);
#59240=EDGE_CURVE('',#44653,#44715,#24302,.T.);
#59241=EDGE_CURVE('',#44715,#44716,#24303,.T.);
#59242=EDGE_CURVE('',#44716,#44717,#24304,.T.);
#59243=EDGE_CURVE('',#44717,#44718,#24305,.T.);
#59244=EDGE_CURVE('',#44719,#44718,#24306,.T.);
#59245=EDGE_CURVE('',#44713,#44719,#24307,.T.);
#59246=EDGE_CURVE('',#44718,#44720,#24308,.T.);
#59247=EDGE_CURVE('',#44721,#44720,#24309,.T.);
#59248=EDGE_CURVE('',#44719,#44721,#24310,.T.);
#59249=EDGE_CURVE('',#44720,#44722,#24311,.T.);
#59250=EDGE_CURVE('',#44722,#44723,#24312,.T.);
#59251=EDGE_CURVE('',#44723,#44724,#24313,.T.);
#59252=EDGE_CURVE('',#44724,#44656,#24314,.T.);
#59253=EDGE_CURVE('',#44721,#44714,#24315,.T.);
#59254=EDGE_CURVE('',#44725,#44726,#24316,.T.);
#59255=EDGE_CURVE('',#44726,#44722,#36257,.T.);
#59256=EDGE_CURVE('',#44717,#44725,#36258,.T.);
#59257=EDGE_CURVE('',#44706,#44690,#36259,.T.);
#59258=EDGE_CURVE('',#44691,#44703,#36260,.T.);
#59259=EDGE_CURVE('',#44692,#44702,#36261,.T.);
#59260=EDGE_CURVE('',#44707,#44689,#36262,.T.);
#59261=EDGE_CURVE('',#44685,#44697,#36263,.T.);
#59262=EDGE_CURVE('',#44694,#44688,#36264,.T.);
#59263=EDGE_CURVE('',#44686,#44700,#36265,.T.);
#59264=EDGE_CURVE('',#44695,#44687,#36266,.T.);
#59265=EDGE_CURVE('',#44704,#44726,#36267,.T.);
#59266=EDGE_CURVE('',#44722,#44710,#36268,.T.);
#59267=EDGE_CURVE('',#44723,#44705,#36269,.T.);
#59268=EDGE_CURVE('',#44701,#44725,#36270,.T.);
#59269=EDGE_CURVE('',#44724,#44708,#36271,.T.);
#59270=EDGE_CURVE('',#44712,#44717,#36272,.T.);
#59271=EDGE_CURVE('',#44656,#44709,#36273,.T.);
#59272=EDGE_CURVE('',#44698,#44716,#36274,.T.);
#59273=EDGE_CURVE('',#44651,#44693,#36275,.T.);
#59274=EDGE_CURVE('',#44699,#44715,#36276,.T.);
#59275=EDGE_CURVE('',#44652,#44696,#36277,.T.);
#59276=EDGE_CURVE('',#44711,#44653,#36278,.T.);
#59277=EDGE_CURVE('',#44727,#44728,#24317,.T.);
#59278=EDGE_CURVE('',#44729,#44727,#24318,.T.);
#59279=EDGE_CURVE('',#44730,#44729,#24319,.T.);
#59280=EDGE_CURVE('',#44728,#44730,#24320,.T.);
#59281=EDGE_CURVE('',#44731,#44728,#24321,.T.);
#59282=EDGE_CURVE('',#44732,#44731,#24322,.T.);
#59283=EDGE_CURVE('',#44732,#44727,#24323,.T.);
#59284=EDGE_CURVE('',#44733,#44730,#24324,.T.);
#59285=EDGE_CURVE('',#44731,#44733,#24325,.T.);
#59286=EDGE_CURVE('',#44734,#44729,#24326,.T.);
#59287=EDGE_CURVE('',#44733,#44734,#24327,.T.);
#59288=EDGE_CURVE('',#44734,#44732,#24328,.T.);
#59289=EDGE_CURVE('',#44672,#44661,#24329,.T.);
#59290=EDGE_CURVE('',#44662,#44671,#24330,.T.);
#87733=ORIENTED_EDGE('',*,*,#59145,.F.);
#87734=ORIENTED_EDGE('',*,*,#59146,.F.);
#87735=ORIENTED_EDGE('',*,*,#59147,.F.);
#87736=ORIENTED_EDGE('',*,*,#59148,.F.);
#87737=ORIENTED_EDGE('',*,*,#59149,.T.);
#87738=ORIENTED_EDGE('',*,*,#59150,.T.);
#87739=ORIENTED_EDGE('',*,*,#59151,.F.);
#87740=ORIENTED_EDGE('',*,*,#59152,.F.);
#87741=ORIENTED_EDGE('',*,*,#59153,.F.);
#87742=ORIENTED_EDGE('',*,*,#59154,.T.);
#87743=ORIENTED_EDGE('',*,*,#59155,.T.);
#87744=ORIENTED_EDGE('',*,*,#59156,.T.);
#87745=ORIENTED_EDGE('',*,*,#59157,.T.);
#87746=ORIENTED_EDGE('',*,*,#59158,.F.);
#87747=ORIENTED_EDGE('',*,*,#59159,.T.);
#87748=ORIENTED_EDGE('',*,*,#59146,.T.);
#87749=ORIENTED_EDGE('',*,*,#59160,.F.);
#87750=ORIENTED_EDGE('',*,*,#59161,.F.);
#87751=ORIENTED_EDGE('',*,*,#59162,.T.);
#87752=ORIENTED_EDGE('',*,*,#59163,.T.);
#87753=ORIENTED_EDGE('',*,*,#59164,.T.);
#87754=ORIENTED_EDGE('',*,*,#59165,.F.);
#87755=ORIENTED_EDGE('',*,*,#59166,.T.);
#87756=ORIENTED_EDGE('',*,*,#59167,.T.);
#87757=ORIENTED_EDGE('',*,*,#59168,.T.);
#87758=ORIENTED_EDGE('',*,*,#59169,.F.);
#87759=ORIENTED_EDGE('',*,*,#59170,.T.);
#87760=ORIENTED_EDGE('',*,*,#59148,.T.);
#87761=ORIENTED_EDGE('',*,*,#59171,.F.);
#87762=ORIENTED_EDGE('',*,*,#59172,.F.);
#87763=ORIENTED_EDGE('',*,*,#59173,.T.);
#87764=ORIENTED_EDGE('',*,*,#59174,.T.);
#87765=ORIENTED_EDGE('',*,*,#59175,.T.);
#87766=ORIENTED_EDGE('',*,*,#59176,.F.);
#87767=ORIENTED_EDGE('',*,*,#59177,.T.);
#87768=ORIENTED_EDGE('',*,*,#59178,.T.);
#87769=ORIENTED_EDGE('',*,*,#59179,.T.);
#87770=ORIENTED_EDGE('',*,*,#59180,.T.);
#87771=ORIENTED_EDGE('',*,*,#59181,.T.);
#87772=ORIENTED_EDGE('',*,*,#59182,.T.);
#87773=ORIENTED_EDGE('',*,*,#59183,.T.);
#87774=ORIENTED_EDGE('',*,*,#59184,.T.);
#87775=ORIENTED_EDGE('',*,*,#59185,.T.);
#87776=ORIENTED_EDGE('',*,*,#59186,.T.);
#87777=ORIENTED_EDGE('',*,*,#59187,.T.);
#87778=ORIENTED_EDGE('',*,*,#59188,.T.);
#87779=ORIENTED_EDGE('',*,*,#59189,.T.);
#87780=ORIENTED_EDGE('',*,*,#59190,.T.);
#87781=ORIENTED_EDGE('',*,*,#59191,.T.);
#87782=ORIENTED_EDGE('',*,*,#59192,.T.);
#87783=ORIENTED_EDGE('',*,*,#59193,.T.);
#87784=ORIENTED_EDGE('',*,*,#59194,.T.);
#87785=ORIENTED_EDGE('',*,*,#59195,.T.);
#87786=ORIENTED_EDGE('',*,*,#59196,.T.);
#87787=ORIENTED_EDGE('',*,*,#59197,.T.);
#87788=ORIENTED_EDGE('',*,*,#59198,.T.);
#87789=ORIENTED_EDGE('',*,*,#59199,.T.);
#87790=ORIENTED_EDGE('',*,*,#59200,.T.);
#87791=ORIENTED_EDGE('',*,*,#59201,.T.);
#87792=ORIENTED_EDGE('',*,*,#59202,.T.);
#87793=ORIENTED_EDGE('',*,*,#59203,.T.);
#87794=ORIENTED_EDGE('',*,*,#59204,.T.);
#87795=ORIENTED_EDGE('',*,*,#59205,.T.);
#87796=ORIENTED_EDGE('',*,*,#59206,.T.);
#87797=ORIENTED_EDGE('',*,*,#59207,.T.);
#87798=ORIENTED_EDGE('',*,*,#59208,.T.);
#87799=ORIENTED_EDGE('',*,*,#59157,.F.);
#87800=ORIENTED_EDGE('',*,*,#59209,.T.);
#87801=ORIENTED_EDGE('',*,*,#59173,.F.);
#87802=ORIENTED_EDGE('',*,*,#59210,.F.);
#87803=ORIENTED_EDGE('',*,*,#59168,.F.);
#87804=ORIENTED_EDGE('',*,*,#59211,.T.);
#87805=ORIENTED_EDGE('',*,*,#59162,.F.);
#87806=ORIENTED_EDGE('',*,*,#59212,.F.);
#87807=ORIENTED_EDGE('',*,*,#59164,.F.);
#87808=ORIENTED_EDGE('',*,*,#59213,.T.);
#87809=ORIENTED_EDGE('',*,*,#59155,.F.);
#87810=ORIENTED_EDGE('',*,*,#59214,.F.);
#87811=ORIENTED_EDGE('',*,*,#59175,.F.);
#87812=ORIENTED_EDGE('',*,*,#59215,.T.);
#87813=ORIENTED_EDGE('',*,*,#59166,.F.);
#87814=ORIENTED_EDGE('',*,*,#59216,.F.);
#87815=ORIENTED_EDGE('',*,*,#59217,.F.);
#87816=ORIENTED_EDGE('',*,*,#59213,.F.);
#87817=ORIENTED_EDGE('',*,*,#59218,.F.);
#87818=ORIENTED_EDGE('',*,*,#59182,.F.);
#87819=ORIENTED_EDGE('',*,*,#59218,.T.);
#87820=ORIENTED_EDGE('',*,*,#59163,.F.);
#87821=ORIENTED_EDGE('',*,*,#59219,.F.);
#87822=ORIENTED_EDGE('',*,*,#59183,.F.);
#87823=ORIENTED_EDGE('',*,*,#59217,.T.);
#87824=ORIENTED_EDGE('',*,*,#59181,.F.);
#87825=ORIENTED_EDGE('',*,*,#59220,.F.);
#87826=ORIENTED_EDGE('',*,*,#59156,.F.);
#87827=ORIENTED_EDGE('',*,*,#59219,.T.);
#87828=ORIENTED_EDGE('',*,*,#59211,.F.);
#87829=ORIENTED_EDGE('',*,*,#59221,.F.);
#87830=ORIENTED_EDGE('',*,*,#59184,.F.);
#87831=ORIENTED_EDGE('',*,*,#59220,.T.);
#87832=ORIENTED_EDGE('',*,*,#59180,.F.);
#87833=ORIENTED_EDGE('',*,*,#59222,.F.);
#87834=ORIENTED_EDGE('',*,*,#59209,.F.);
#87835=ORIENTED_EDGE('',*,*,#59221,.T.);
#87836=ORIENTED_EDGE('',*,*,#59167,.F.);
#87837=ORIENTED_EDGE('',*,*,#59223,.F.);
#87838=ORIENTED_EDGE('',*,*,#59177,.F.);
#87839=ORIENTED_EDGE('',*,*,#59222,.T.);
#87840=ORIENTED_EDGE('',*,*,#59179,.F.);
#87841=ORIENTED_EDGE('',*,*,#59224,.F.);
#87842=ORIENTED_EDGE('',*,*,#59174,.F.);
#87843=ORIENTED_EDGE('',*,*,#59223,.T.);
#87844=ORIENTED_EDGE('',*,*,#59215,.F.);
#87845=ORIENTED_EDGE('',*,*,#59224,.T.);
#87846=ORIENTED_EDGE('',*,*,#59178,.F.);
#87847=ORIENTED_EDGE('',*,*,#59207,.F.);
#87848=ORIENTED_EDGE('',*,*,#59225,.T.);
#87849=ORIENTED_EDGE('',*,*,#59193,.F.);
#87850=ORIENTED_EDGE('',*,*,#59226,.T.);
#87851=ORIENTED_EDGE('',*,*,#59227,.T.);
#87852=ORIENTED_EDGE('',*,*,#59203,.F.);
#87853=ORIENTED_EDGE('',*,*,#59228,.T.);
#87854=ORIENTED_EDGE('',*,*,#59205,.F.);
#87855=ORIENTED_EDGE('',*,*,#59229,.T.);
#87856=ORIENTED_EDGE('',*,*,#59230,.T.);
#87857=ORIENTED_EDGE('',*,*,#59195,.F.);
#87858=ORIENTED_EDGE('',*,*,#59231,.T.);
#87859=ORIENTED_EDGE('',*,*,#59199,.F.);
#87860=ORIENTED_EDGE('',*,*,#59232,.T.);
#87861=ORIENTED_EDGE('',*,*,#59233,.T.);
#87862=ORIENTED_EDGE('',*,*,#59197,.F.);
#87863=ORIENTED_EDGE('',*,*,#59234,.T.);
#87864=ORIENTED_EDGE('',*,*,#59201,.F.);
#87865=ORIENTED_EDGE('',*,*,#59235,.T.);
#87866=ORIENTED_EDGE('',*,*,#59236,.T.);
#87867=ORIENTED_EDGE('',*,*,#59152,.T.);
#87868=ORIENTED_EDGE('',*,*,#59237,.F.);
#87869=ORIENTED_EDGE('',*,*,#59238,.F.);
#87870=ORIENTED_EDGE('',*,*,#59239,.T.);
#87871=ORIENTED_EDGE('',*,*,#59151,.T.);
#87872=ORIENTED_EDGE('',*,*,#59240,.T.);
#87873=ORIENTED_EDGE('',*,*,#59241,.T.);
#87874=ORIENTED_EDGE('',*,*,#59242,.T.);
#87875=ORIENTED_EDGE('',*,*,#59243,.T.);
#87876=ORIENTED_EDGE('',*,*,#59244,.F.);
#87877=ORIENTED_EDGE('',*,*,#59245,.F.);
#87878=ORIENTED_EDGE('',*,*,#59237,.T.);
#87879=ORIENTED_EDGE('',*,*,#59246,.T.);
#87880=ORIENTED_EDGE('',*,*,#59247,.F.);
#87881=ORIENTED_EDGE('',*,*,#59248,.F.);
#87882=ORIENTED_EDGE('',*,*,#59244,.T.);
#87883=ORIENTED_EDGE('',*,*,#59249,.T.);
#87884=ORIENTED_EDGE('',*,*,#59250,.T.);
#87885=ORIENTED_EDGE('',*,*,#59251,.T.);
#87886=ORIENTED_EDGE('',*,*,#59252,.T.);
#87887=ORIENTED_EDGE('',*,*,#59153,.T.);
#87888=ORIENTED_EDGE('',*,*,#59239,.F.);
#87889=ORIENTED_EDGE('',*,*,#59253,.F.);
#87890=ORIENTED_EDGE('',*,*,#59247,.T.);
#87891=ORIENTED_EDGE('',*,*,#59254,.T.);
#87892=ORIENTED_EDGE('',*,*,#59255,.T.);
#87893=ORIENTED_EDGE('',*,*,#59249,.F.);
#87894=ORIENTED_EDGE('',*,*,#59246,.F.);
#87895=ORIENTED_EDGE('',*,*,#59243,.F.);
#87896=ORIENTED_EDGE('',*,*,#59256,.T.);
#87897=ORIENTED_EDGE('',*,*,#59257,.F.);
#87898=ORIENTED_EDGE('',*,*,#59228,.F.);
#87899=ORIENTED_EDGE('',*,*,#59258,.F.);
#87900=ORIENTED_EDGE('',*,*,#59190,.F.);
#87901=ORIENTED_EDGE('',*,*,#59258,.T.);
#87902=ORIENTED_EDGE('',*,*,#59202,.F.);
#87903=ORIENTED_EDGE('',*,*,#59259,.F.);
#87904=ORIENTED_EDGE('',*,*,#59191,.F.);
#87905=ORIENTED_EDGE('',*,*,#59257,.T.);
#87906=ORIENTED_EDGE('',*,*,#59189,.F.);
#87907=ORIENTED_EDGE('',*,*,#59260,.F.);
#87908=ORIENTED_EDGE('',*,*,#59206,.F.);
#87909=ORIENTED_EDGE('',*,*,#59259,.T.);
#87910=ORIENTED_EDGE('',*,*,#59234,.F.);
#87911=ORIENTED_EDGE('',*,*,#59261,.F.);
#87912=ORIENTED_EDGE('',*,*,#59192,.F.);
#87913=ORIENTED_EDGE('',*,*,#59260,.T.);
#87914=ORIENTED_EDGE('',*,*,#59188,.F.);
#87915=ORIENTED_EDGE('',*,*,#59262,.F.);
#87916=ORIENTED_EDGE('',*,*,#59225,.F.);
#87917=ORIENTED_EDGE('',*,*,#59261,.T.);
#87918=ORIENTED_EDGE('',*,*,#59200,.F.);
#87919=ORIENTED_EDGE('',*,*,#59263,.F.);
#87920=ORIENTED_EDGE('',*,*,#59185,.F.);
#87921=ORIENTED_EDGE('',*,*,#59262,.T.);
#87922=ORIENTED_EDGE('',*,*,#59187,.F.);
#87923=ORIENTED_EDGE('',*,*,#59264,.F.);
#87924=ORIENTED_EDGE('',*,*,#59194,.F.);
#87925=ORIENTED_EDGE('',*,*,#59263,.T.);
#87926=ORIENTED_EDGE('',*,*,#59231,.F.);
#87927=ORIENTED_EDGE('',*,*,#59264,.T.);
#87928=ORIENTED_EDGE('',*,*,#59186,.F.);
#87929=ORIENTED_EDGE('',*,*,#59265,.F.);
#87930=ORIENTED_EDGE('',*,*,#59230,.F.);
#87931=ORIENTED_EDGE('',*,*,#59266,.F.);
#87932=ORIENTED_EDGE('',*,*,#59255,.F.);
#87933=ORIENTED_EDGE('',*,*,#59266,.T.);
#87934=ORIENTED_EDGE('',*,*,#59229,.F.);
#87935=ORIENTED_EDGE('',*,*,#59267,.F.);
#87936=ORIENTED_EDGE('',*,*,#59250,.F.);
#87937=ORIENTED_EDGE('',*,*,#59265,.T.);
#87938=ORIENTED_EDGE('',*,*,#59254,.F.);
#87939=ORIENTED_EDGE('',*,*,#59268,.F.);
#87940=ORIENTED_EDGE('',*,*,#59204,.F.);
#87941=ORIENTED_EDGE('',*,*,#59267,.T.);
#87942=ORIENTED_EDGE('',*,*,#59208,.F.);
#87943=ORIENTED_EDGE('',*,*,#59269,.F.);
#87944=ORIENTED_EDGE('',*,*,#59251,.F.);
#87945=ORIENTED_EDGE('',*,*,#59268,.T.);
#87946=ORIENTED_EDGE('',*,*,#59256,.F.);
#87947=ORIENTED_EDGE('',*,*,#59270,.F.);
#87948=ORIENTED_EDGE('',*,*,#59235,.F.);
#87949=ORIENTED_EDGE('',*,*,#59269,.T.);
#87950=ORIENTED_EDGE('',*,*,#59227,.F.);
#87951=ORIENTED_EDGE('',*,*,#59271,.F.);
#87952=ORIENTED_EDGE('',*,*,#59252,.F.);
#87953=ORIENTED_EDGE('',*,*,#59270,.T.);
#87954=ORIENTED_EDGE('',*,*,#59242,.F.);
#87955=ORIENTED_EDGE('',*,*,#59272,.F.);
#87956=ORIENTED_EDGE('',*,*,#59236,.F.);
#87957=ORIENTED_EDGE('',*,*,#59271,.T.);
#87958=ORIENTED_EDGE('',*,*,#59226,.F.);
#87959=ORIENTED_EDGE('',*,*,#59273,.F.);
#87960=ORIENTED_EDGE('',*,*,#59154,.F.);
#87961=ORIENTED_EDGE('',*,*,#59272,.T.);
#87962=ORIENTED_EDGE('',*,*,#59241,.F.);
#87963=ORIENTED_EDGE('',*,*,#59274,.F.);
#87964=ORIENTED_EDGE('',*,*,#59198,.F.);
#87965=ORIENTED_EDGE('',*,*,#59273,.T.);
#87966=ORIENTED_EDGE('',*,*,#59196,.F.);
#87967=ORIENTED_EDGE('',*,*,#59275,.F.);
#87968=ORIENTED_EDGE('',*,*,#59149,.F.);
#87969=ORIENTED_EDGE('',*,*,#59274,.T.);
#87970=ORIENTED_EDGE('',*,*,#59240,.F.);
#87971=ORIENTED_EDGE('',*,*,#59276,.F.);
#87972=ORIENTED_EDGE('',*,*,#59232,.F.);
#87973=ORIENTED_EDGE('',*,*,#59275,.T.);
#87974=ORIENTED_EDGE('',*,*,#59233,.F.);
#87975=ORIENTED_EDGE('',*,*,#59276,.T.);
#87976=ORIENTED_EDGE('',*,*,#59150,.F.);
#87977=ORIENTED_EDGE('',*,*,#59277,.F.);
#87978=ORIENTED_EDGE('',*,*,#59278,.F.);
#87979=ORIENTED_EDGE('',*,*,#59279,.F.);
#87980=ORIENTED_EDGE('',*,*,#59280,.F.);
#87981=ORIENTED_EDGE('',*,*,#59253,.T.);
#87982=ORIENTED_EDGE('',*,*,#59238,.T.);
#87983=ORIENTED_EDGE('',*,*,#59245,.T.);
#87984=ORIENTED_EDGE('',*,*,#59248,.T.);
#87985=ORIENTED_EDGE('',*,*,#59277,.T.);
#87986=ORIENTED_EDGE('',*,*,#59281,.F.);
#87987=ORIENTED_EDGE('',*,*,#59282,.F.);
#87988=ORIENTED_EDGE('',*,*,#59283,.T.);
#87989=ORIENTED_EDGE('',*,*,#59280,.T.);
#87990=ORIENTED_EDGE('',*,*,#59284,.F.);
#87991=ORIENTED_EDGE('',*,*,#59285,.F.);
#87992=ORIENTED_EDGE('',*,*,#59281,.T.);
#87993=ORIENTED_EDGE('',*,*,#59279,.T.);
#87994=ORIENTED_EDGE('',*,*,#59286,.F.);
#87995=ORIENTED_EDGE('',*,*,#59287,.F.);
#87996=ORIENTED_EDGE('',*,*,#59284,.T.);
#87997=ORIENTED_EDGE('',*,*,#59278,.T.);
#87998=ORIENTED_EDGE('',*,*,#59283,.F.);
#87999=ORIENTED_EDGE('',*,*,#59288,.F.);
#88000=ORIENTED_EDGE('',*,*,#59286,.T.);
#88001=ORIENTED_EDGE('',*,*,#59282,.T.);
#88002=ORIENTED_EDGE('',*,*,#59285,.T.);
#88003=ORIENTED_EDGE('',*,*,#59287,.T.);
#88004=ORIENTED_EDGE('',*,*,#59288,.T.);
#88005=ORIENTED_EDGE('',*,*,#59147,.T.);
#88006=ORIENTED_EDGE('',*,*,#59159,.F.);
#88007=ORIENTED_EDGE('',*,*,#59289,.F.);
#88008=ORIENTED_EDGE('',*,*,#59171,.T.);
#88009=ORIENTED_EDGE('',*,*,#59210,.T.);
#88010=ORIENTED_EDGE('',*,*,#59176,.T.);
#88011=ORIENTED_EDGE('',*,*,#59216,.T.);
#88012=ORIENTED_EDGE('',*,*,#59172,.T.);
#88013=ORIENTED_EDGE('',*,*,#59289,.T.);
#88014=ORIENTED_EDGE('',*,*,#59158,.T.);
#88015=ORIENTED_EDGE('',*,*,#59145,.T.);
#88016=ORIENTED_EDGE('',*,*,#59170,.F.);
#88017=ORIENTED_EDGE('',*,*,#59290,.F.);
#88018=ORIENTED_EDGE('',*,*,#59160,.T.);
#88019=ORIENTED_EDGE('',*,*,#59214,.T.);
#88020=ORIENTED_EDGE('',*,*,#59161,.T.);
#88021=ORIENTED_EDGE('',*,*,#59290,.T.);
#88022=ORIENTED_EDGE('',*,*,#59169,.T.);
#88023=ORIENTED_EDGE('',*,*,#59212,.T.);
#88024=ORIENTED_EDGE('',*,*,#59165,.T.);
#92427=CYLINDRICAL_SURFACE('',#110897,5.);
#92428=CYLINDRICAL_SURFACE('',#110900,5.);
#92429=CYLINDRICAL_SURFACE('',#110903,5.);
#92430=CYLINDRICAL_SURFACE('',#110906,5.);
#92431=CYLINDRICAL_SURFACE('',#110911,3.);
#92432=CYLINDRICAL_SURFACE('',#110913,3.);
#92433=CYLINDRICAL_SURFACE('',#110917,3.);
#92434=CYLINDRICAL_SURFACE('',#110919,3.);
#92435=CYLINDRICAL_SURFACE('',#110921,5.);
#92436=CYLINDRICAL_SURFACE('',#110924,5.);
#92437=CYLINDRICAL_SURFACE('',#110927,5.);
#92438=CYLINDRICAL_SURFACE('',#110930,5.);
#92439=CYLINDRICAL_SURFACE('',#110943,5.);
#92440=CYLINDRICAL_SURFACE('',#110945,5.);
#92441=CYLINDRICAL_SURFACE('',#110951,5.);
#92442=CYLINDRICAL_SURFACE('',#110953,5.);
#92443=CYLINDRICAL_SURFACE('',#110960,5.);
#92444=CYLINDRICAL_SURFACE('',#110962,5.);
#92445=CYLINDRICAL_SURFACE('',#110970,5.);
#92446=CYLINDRICAL_SURFACE('',#110972,5.);
#98235=ADVANCED_FACE('',(#13262),#7328,.F.);
#98236=ADVANCED_FACE('',(#13263),#7329,.F.);
#98237=ADVANCED_FACE('',(#13264),#7330,.F.);
#98238=ADVANCED_FACE('',(#13265),#7331,.F.);
#98239=ADVANCED_FACE('',(#13266),#7332,.F.);
#98240=ADVANCED_FACE('',(#13267),#7333,.F.);
#98241=ADVANCED_FACE('',(#13268,#6442),#7334,.T.);
#98242=ADVANCED_FACE('',(#13269),#7335,.F.);
#98243=ADVANCED_FACE('',(#13270),#7336,.F.);
#98244=ADVANCED_FACE('',(#13271),#7337,.F.);
#98245=ADVANCED_FACE('',(#13272),#7338,.F.);
#98246=ADVANCED_FACE('',(#13273),#92427,.T.);
#98247=ADVANCED_FACE('',(#13274),#92428,.T.);
#98248=ADVANCED_FACE('',(#13275),#92429,.T.);
#98249=ADVANCED_FACE('',(#13276),#92430,.T.);
#98250=ADVANCED_FACE('',(#13277),#4057,.F.);
#98251=ADVANCED_FACE('',(#13278),#92431,.T.);
#98252=ADVANCED_FACE('',(#13279),#92432,.T.);
#98253=ADVANCED_FACE('',(#13280),#4058,.F.);
#98254=ADVANCED_FACE('',(#13281),#4059,.F.);
#98255=ADVANCED_FACE('',(#13282),#92433,.T.);
#98256=ADVANCED_FACE('',(#13283),#92434,.T.);
#98257=ADVANCED_FACE('',(#13284),#4060,.F.);
#98258=ADVANCED_FACE('',(#13285),#92435,.T.);
#98259=ADVANCED_FACE('',(#13286),#92436,.T.);
#98260=ADVANCED_FACE('',(#13287),#92437,.T.);
#98261=ADVANCED_FACE('',(#13288),#92438,.T.);
#98262=ADVANCED_FACE('',(#13289),#7339,.F.);
#98263=ADVANCED_FACE('',(#13290),#7340,.F.);
#98264=ADVANCED_FACE('',(#13291),#7341,.F.);
#98265=ADVANCED_FACE('',(#13292),#7342,.F.);
#98266=ADVANCED_FACE('',(#13293),#7343,.F.);
#98267=ADVANCED_FACE('',(#13294),#6314,.F.);
#98268=ADVANCED_FACE('',(#13295),#92439,.F.);
#98269=ADVANCED_FACE('',(#13296),#92440,.F.);
#98270=ADVANCED_FACE('',(#13297),#6315,.F.);
#98271=ADVANCED_FACE('',(#13298),#6316,.F.);
#98272=ADVANCED_FACE('',(#13299),#92441,.F.);
#98273=ADVANCED_FACE('',(#13300),#92442,.F.);
#98274=ADVANCED_FACE('',(#13301),#6317,.F.);
#98275=ADVANCED_FACE('',(#13302),#6318,.F.);
#98276=ADVANCED_FACE('',(#13303),#4061,.F.);
#98277=ADVANCED_FACE('',(#13304),#92443,.F.);
#98278=ADVANCED_FACE('',(#13305),#92444,.F.);
#98279=ADVANCED_FACE('',(#13306),#6319,.F.);
#98280=ADVANCED_FACE('',(#13307),#4062,.F.);
#98281=ADVANCED_FACE('',(#13308),#4063,.F.);
#98282=ADVANCED_FACE('',(#13309),#6320,.F.);
#98283=ADVANCED_FACE('',(#13310),#92445,.F.);
#98284=ADVANCED_FACE('',(#13311),#92446,.F.);
#98285=ADVANCED_FACE('',(#13312),#4064,.F.);
#98286=ADVANCED_FACE('',(#13313),#6321,.F.);
#98287=ADVANCED_FACE('',(#13314,#6443),#7344,.F.);
#98288=ADVANCED_FACE('',(#13315),#7345,.F.);
#98289=ADVANCED_FACE('',(#13316),#7346,.F.);
#98290=ADVANCED_FACE('',(#13317),#7347,.F.);
#98291=ADVANCED_FACE('',(#13318),#7348,.F.);
#98292=ADVANCED_FACE('',(#13319),#7349,.T.);
#98293=ADVANCED_FACE('',(#13320),#7350,.F.);
#98294=ADVANCED_FACE('',(#13321),#7351,.T.);
#98295=ADVANCED_FACE('',(#13322),#7352,.F.);
#98296=ADVANCED_FACE('',(#13323),#7353,.T.);
#98724=CLOSED_SHELL('',(#98235,#98236,#98237,#98238,#98239,#98240,#98241,
#98242,#98243,#98244,#98245,#98246,#98247,#98248,#98249,#98250,#98251,#98252,
#98253,#98254,#98255,#98256,#98257,#98258,#98259,#98260,#98261,#98262,#98263,
#98264,#98265,#98266,#98267,#98268,#98269,#98270,#98271,#98272,#98273,#98274,
#98275,#98276,#98277,#98278,#98279,#98280,#98281,#98282,#98283,#98284,#98285,
#98286,#98287,#98288,#98289,#98290,#98291,#98292,#98293,#98294,#98295,#98296));
#110875=AXIS2_PLACEMENT_3D('',#273741,#140106,#140107);
#110876=AXIS2_PLACEMENT_3D('',#273742,#140108,#140109);
#110877=AXIS2_PLACEMENT_3D('',#273751,#140114,#140115);
#110878=AXIS2_PLACEMENT_3D('',#273756,#140117,#140118);
#110879=AXIS2_PLACEMENT_3D('',#273763,#140122,#140123);
#110880=AXIS2_PLACEMENT_3D('',#273764,#140124,#140125);
#110881=AXIS2_PLACEMENT_3D('',#273778,#140133,#140134);
#110882=AXIS2_PLACEMENT_3D('',#273787,#140139,#140140);
#110883=AXIS2_PLACEMENT_3D('',#273801,#140148,#140149);
#110884=AXIS2_PLACEMENT_3D('',#273810,#140154,#140155);
#110885=AXIS2_PLACEMENT_3D('',#273815,#140157,#140158);
#110886=AXIS2_PLACEMENT_3D('',#273819,#140160,#140161);
#110887=AXIS2_PLACEMENT_3D('',#273823,#140163,#140164);
#110888=AXIS2_PLACEMENT_3D('',#273826,#140166,#140167);
#110889=AXIS2_PLACEMENT_3D('',#273831,#140169,#140170);
#110890=AXIS2_PLACEMENT_3D('',#273835,#140172,#140173);
#110891=AXIS2_PLACEMENT_3D('',#273839,#140175,#140176);
#110892=AXIS2_PLACEMENT_3D('',#273842,#140178,#140179);
#110893=AXIS2_PLACEMENT_3D('',#273843,#140180,#140181);
#110894=AXIS2_PLACEMENT_3D('',#273852,#140186,#140187);
#110895=AXIS2_PLACEMENT_3D('',#273861,#140192,#140193);
#110896=AXIS2_PLACEMENT_3D('',#273870,#140198,#140199);
#110897=AXIS2_PLACEMENT_3D('',#273879,#140204,#140205);
#110898=AXIS2_PLACEMENT_3D('',#273880,#140206,#140207);
#110899=AXIS2_PLACEMENT_3D('',#273881,#140208,#140209);
#110900=AXIS2_PLACEMENT_3D('',#273882,#140210,#140211);
#110901=AXIS2_PLACEMENT_3D('',#273883,#140212,#140213);
#110902=AXIS2_PLACEMENT_3D('',#273884,#140214,#140215);
#110903=AXIS2_PLACEMENT_3D('',#273885,#140216,#140217);
#110904=AXIS2_PLACEMENT_3D('',#273886,#140218,#140219);
#110905=AXIS2_PLACEMENT_3D('',#273887,#140220,#140221);
#110906=AXIS2_PLACEMENT_3D('',#273888,#140222,#140223);
#110907=AXIS2_PLACEMENT_3D('',#273889,#140224,#140225);
#110908=AXIS2_PLACEMENT_3D('',#273890,#140226,#140227);
#110909=AXIS2_PLACEMENT_3D('',#273900,#140228,#140229);
#110910=AXIS2_PLACEMENT_3D('',#273901,#140230,#140231);
#110911=AXIS2_PLACEMENT_3D('',#273902,#140232,#140233);
#110912=AXIS2_PLACEMENT_3D('',#273903,#140234,#140235);
#110913=AXIS2_PLACEMENT_3D('',#273904,#140236,#140237);
#110914=AXIS2_PLACEMENT_3D('',#273905,#140238,#140239);
#110915=AXIS2_PLACEMENT_3D('',#273915,#140240,#140241);
#110916=AXIS2_PLACEMENT_3D('',#273925,#140242,#140243);
#110917=AXIS2_PLACEMENT_3D('',#273926,#140244,#140245);
#110918=AXIS2_PLACEMENT_3D('',#273927,#140246,#140247);
#110919=AXIS2_PLACEMENT_3D('',#273928,#140248,#140249);
#110920=AXIS2_PLACEMENT_3D('',#273929,#140250,#140251);
#110921=AXIS2_PLACEMENT_3D('',#273939,#140252,#140253);
#110922=AXIS2_PLACEMENT_3D('',#273940,#140254,#140255);
#110923=AXIS2_PLACEMENT_3D('',#273942,#140256,#140257);
#110924=AXIS2_PLACEMENT_3D('',#273953,#140258,#140259);
#110925=AXIS2_PLACEMENT_3D('',#273954,#140260,#140261);
#110926=AXIS2_PLACEMENT_3D('',#273966,#140262,#140263);
#110927=AXIS2_PLACEMENT_3D('',#273967,#140264,#140265);
#110928=AXIS2_PLACEMENT_3D('',#273968,#140266,#140267);
#110929=AXIS2_PLACEMENT_3D('',#273980,#140268,#140269);
#110930=AXIS2_PLACEMENT_3D('',#273981,#140270,#140271);
#110931=AXIS2_PLACEMENT_3D('',#273982,#140272,#140273);
#110932=AXIS2_PLACEMENT_3D('',#273984,#140274,#140275);
#110933=AXIS2_PLACEMENT_3D('',#273995,#140276,#140277);
#110934=AXIS2_PLACEMENT_3D('',#274001,#140281,#140282);
#110935=AXIS2_PLACEMENT_3D('',#274013,#140289,#140290);
#110936=AXIS2_PLACEMENT_3D('',#274019,#140294,#140295);
#110937=AXIS2_PLACEMENT_3D('',#274028,#140301,#140302);
#110938=AXIS2_PLACEMENT_3D('',#274032,#140304,#140305);
#110939=AXIS2_PLACEMENT_3D('',#274033,#140306,#140307);
#110940=AXIS2_PLACEMENT_3D('',#274034,#140308,#140309);
#110941=AXIS2_PLACEMENT_3D('',#274035,#140310,#140311);
#110942=AXIS2_PLACEMENT_3D('',#274036,#140312,#140313);
#110943=AXIS2_PLACEMENT_3D('',#274037,#140314,#140315);
#110944=AXIS2_PLACEMENT_3D('',#274038,#140316,#140317);
#110945=AXIS2_PLACEMENT_3D('',#274039,#140318,#140319);
#110946=AXIS2_PLACEMENT_3D('',#274040,#140320,#140321);
#110947=AXIS2_PLACEMENT_3D('',#274041,#140322,#140323);
#110948=AXIS2_PLACEMENT_3D('',#274042,#140324,#140325);
#110949=AXIS2_PLACEMENT_3D('',#274043,#140326,#140327);
#110950=AXIS2_PLACEMENT_3D('',#274044,#140328,#140329);
#110951=AXIS2_PLACEMENT_3D('',#274045,#140330,#140331);
#110952=AXIS2_PLACEMENT_3D('',#274046,#140332,#140333);
#110953=AXIS2_PLACEMENT_3D('',#274047,#140334,#140335);
#110954=AXIS2_PLACEMENT_3D('',#274048,#140336,#140337);
#110955=AXIS2_PLACEMENT_3D('',#274049,#140338,#140339);
#110956=AXIS2_PLACEMENT_3D('',#274050,#140340,#140341);
#110957=AXIS2_PLACEMENT_3D('',#274051,#140342,#140343);
#110958=AXIS2_PLACEMENT_3D('',#274052,#140344,#140345);
#110959=AXIS2_PLACEMENT_3D('',#274065,#140346,#140347);
#110960=AXIS2_PLACEMENT_3D('',#274066,#140348,#140349);
#110961=AXIS2_PLACEMENT_3D('',#274067,#140350,#140351);
#110962=AXIS2_PLACEMENT_3D('',#274068,#140352,#140353);
#110963=AXIS2_PLACEMENT_3D('',#274069,#140354,#140355);
#110964=AXIS2_PLACEMENT_3D('',#274070,#140356,#140357);
#110965=AXIS2_PLACEMENT_3D('',#274071,#140358,#140359);
#110966=AXIS2_PLACEMENT_3D('',#274084,#140360,#140361);
#110967=AXIS2_PLACEMENT_3D('',#274097,#140362,#140363);
#110968=AXIS2_PLACEMENT_3D('',#274098,#140364,#140365);
#110969=AXIS2_PLACEMENT_3D('',#274099,#140366,#140367);
#110970=AXIS2_PLACEMENT_3D('',#274100,#140368,#140369);
#110971=AXIS2_PLACEMENT_3D('',#274101,#140370,#140371);
#110972=AXIS2_PLACEMENT_3D('',#274102,#140372,#140373);
#110973=AXIS2_PLACEMENT_3D('',#274103,#140374,#140375);
#110974=AXIS2_PLACEMENT_3D('',#274116,#140376,#140377);
#110975=AXIS2_PLACEMENT_3D('',#274117,#140378,#140379);
#110976=AXIS2_PLACEMENT_3D('',#274118,#140380,#140381);
#110977=AXIS2_PLACEMENT_3D('',#274127,#140386,#140387);
#110978=AXIS2_PLACEMENT_3D('',#274133,#140391,#140392);
#110979=AXIS2_PLACEMENT_3D('',#274137,#140395,#140396);
#110980=AXIS2_PLACEMENT_3D('',#274141,#140399,#140400);
#110981=AXIS2_PLACEMENT_3D('',#274143,#140402,#140403);
#110982=AXIS2_PLACEMENT_3D('',#274144,#140404,#140405);
#110983=AXIS2_PLACEMENT_3D('',#274146,#140407,#140408);
#110984=AXIS2_PLACEMENT_3D('',#274147,#140409,#140410);
#110985=AXIS2_PLACEMENT_3D('',#274149,#140412,#140413);
#140106=DIRECTION('axis',(0.,0.,1.));
#140107=DIRECTION('refdir',(1.,0.,0.));
#140108=DIRECTION('center_axis',(0.,0.,1.));
#140109=DIRECTION('ref_axis',(1.,0.,0.));
#140110=DIRECTION('',(1.,0.,0.));
#140111=DIRECTION('',(0.,-1.,0.));
#140112=DIRECTION('',(-1.,0.,0.));
#140113=DIRECTION('',(0.,1.,0.));
#140114=DIRECTION('center_axis',(0.,0.,1.));
#140115=DIRECTION('ref_axis',(1.,0.,0.));
#140116=DIRECTION('',(0.,1.,0.));
#140117=DIRECTION('center_axis',(0.,0.,1.));
#140118=DIRECTION('ref_axis',(1.,0.,0.));
#140119=DIRECTION('',(-1.,0.,0.));
#140120=DIRECTION('',(0.,1.,0.));
#140121=DIRECTION('',(1.,0.,0.));
#140122=DIRECTION('center_axis',(0.,0.,1.));
#140123=DIRECTION('ref_axis',(1.,0.,0.));
#140124=DIRECTION('center_axis',(1.,0.,0.));
#140125=DIRECTION('ref_axis',(0.,0.,-1.));
#140126=DIRECTION('',(0.,0.,1.));
#140127=DIRECTION('',(0.,1.,0.));
#140128=DIRECTION('',(0.,0.,-1.));
#140129=DIRECTION('',(-4.08120948402688E-16,1.,0.));
#140130=DIRECTION('',(0.,0.,1.));
#140131=DIRECTION('',(0.,0.,1.));
#140132=DIRECTION('',(4.10921029238558E-16,1.,0.));
#140133=DIRECTION('center_axis',(0.,1.,0.));
#140134=DIRECTION('ref_axis',(0.,0.,1.));
#140135=DIRECTION('',(0.,0.,1.));
#140136=DIRECTION('',(-1.,0.,0.));
#140137=DIRECTION('',(0.,0.,-1.));
#140138=DIRECTION('',(-1.,0.,0.));
#140139=DIRECTION('center_axis',(-1.,0.,0.));
#140140=DIRECTION('ref_axis',(0.,0.,1.));
#140141=DIRECTION('',(0.,0.,1.));
#140142=DIRECTION('',(0.,-1.,0.));
#140143=DIRECTION('',(0.,0.,-1.));
#140144=DIRECTION('',(0.,-1.,0.));
#140145=DIRECTION('',(0.,0.,1.));
#140146=DIRECTION('',(0.,0.,1.));
#140147=DIRECTION('',(0.,-1.,0.));
#140148=DIRECTION('center_axis',(0.,-1.,0.));
#140149=DIRECTION('ref_axis',(0.,0.,-1.));
#140150=DIRECTION('',(0.,0.,1.));
#140151=DIRECTION('',(1.,0.,0.));
#140152=DIRECTION('',(0.,0.,-1.));
#140153=DIRECTION('',(1.,0.,0.));
#140154=DIRECTION('center_axis',(0.,0.,1.));
#140155=DIRECTION('ref_axis',(1.,0.,0.));
#140156=DIRECTION('',(0.,1.,0.));
#140157=DIRECTION('center_axis',(0.,0.,1.));
#140158=DIRECTION('ref_axis',(1.,0.,0.));
#140159=DIRECTION('',(-1.,0.,0.));
#140160=DIRECTION('center_axis',(0.,0.,1.));
#140161=DIRECTION('ref_axis',(1.,0.,0.));
#140162=DIRECTION('',(0.,-1.,0.));
#140163=DIRECTION('center_axis',(0.,0.,1.));
#140164=DIRECTION('ref_axis',(1.,0.,0.));
#140165=DIRECTION('',(1.,0.,0.));
#140166=DIRECTION('center_axis',(0.,0.,1.));
#140167=DIRECTION('ref_axis',(1.,0.,0.));
#140168=DIRECTION('',(1.,0.,0.));
#140169=DIRECTION('center_axis',(0.,0.,-1.));
#140170=DIRECTION('ref_axis',(1.,0.,0.));
#140171=DIRECTION('',(0.,-1.,0.));
#140172=DIRECTION('center_axis',(0.,0.,-1.));
#140173=DIRECTION('ref_axis',(1.,0.,0.));
#140174=DIRECTION('',(-1.,0.,0.));
#140175=DIRECTION('center_axis',(0.,0.,-1.));
#140176=DIRECTION('ref_axis',(1.,0.,0.));
#140177=DIRECTION('',(0.,1.,0.));
#140178=DIRECTION('center_axis',(0.,0.,-1.));
#140179=DIRECTION('ref_axis',(1.,0.,0.));
#140180=DIRECTION('center_axis',(-1.,0.,0.));
#140181=DIRECTION('ref_axis',(0.,0.,1.));
#140182=DIRECTION('',(0.,0.,-1.));
#140183=DIRECTION('',(0.,1.,0.));
#140184=DIRECTION('',(0.,0.,1.));
#140185=DIRECTION('',(0.,-1.,0.));
#140186=DIRECTION('center_axis',(0.,-1.,0.));
#140187=DIRECTION('ref_axis',(0.,0.,-1.));
#140188=DIRECTION('',(0.,0.,1.));
#140189=DIRECTION('',(1.,0.,0.));
#140190=DIRECTION('',(0.,0.,-1.));
#140191=DIRECTION('',(-1.,0.,0.));
#140192=DIRECTION('center_axis',(1.,0.,0.));
#140193=DIRECTION('ref_axis',(0.,0.,-1.));
#140194=DIRECTION('',(0.,0.,-1.));
#140195=DIRECTION('',(0.,-1.,0.));
#140196=DIRECTION('',(0.,0.,1.));
#140197=DIRECTION('',(0.,1.,0.));
#140198=DIRECTION('center_axis',(0.,1.,0.));
#140199=DIRECTION('ref_axis',(0.,0.,1.));
#140200=DIRECTION('',(0.,0.,-1.));
#140201=DIRECTION('',(1.,0.,0.));
#140202=DIRECTION('',(0.,0.,1.));
#140203=DIRECTION('',(-1.,0.,0.));
#140204=DIRECTION('center_axis',(0.,0.,-1.));
#140205=DIRECTION('ref_axis',(-1.,0.,0.));
#140206=DIRECTION('center_axis',(0.,0.,-1.));
#140207=DIRECTION('ref_axis',(1.,0.,0.));
#140208=DIRECTION('center_axis',(0.,0.,-1.));
#140209=DIRECTION('ref_axis',(-1.,0.,0.));
#140210=DIRECTION('center_axis',(0.,0.,-1.));
#140211=DIRECTION('ref_axis',(-1.,0.,0.));
#140212=DIRECTION('center_axis',(0.,0.,-1.));
#140213=DIRECTION('ref_axis',(1.,0.,0.));
#140214=DIRECTION('center_axis',(0.,0.,-1.));
#140215=DIRECTION('ref_axis',(-1.,0.,0.));
#140216=DIRECTION('center_axis',(0.,0.,-1.));
#140217=DIRECTION('ref_axis',(-1.,0.,0.));
#140218=DIRECTION('center_axis',(0.,0.,-1.));
#140219=DIRECTION('ref_axis',(1.,0.,0.));
#140220=DIRECTION('center_axis',(0.,0.,-1.));
#140221=DIRECTION('ref_axis',(-1.,0.,0.));
#140222=DIRECTION('center_axis',(0.,0.,-1.));
#140223=DIRECTION('ref_axis',(-1.,0.,0.));
#140224=DIRECTION('center_axis',(0.,0.,-1.));
#140225=DIRECTION('ref_axis',(1.,0.,0.));
#140226=DIRECTION('center_axis',(0.,0.,-1.));
#140227=DIRECTION('ref_axis',(-1.,0.,0.));
#140228=DIRECTION('center_axis',(0.,1.,0.));
#140229=DIRECTION('ref_axis',(0.,0.,1.));
#140230=DIRECTION('center_axis',(1.,0.,0.));
#140231=DIRECTION('ref_axis',(0.,0.,-1.));
#140232=DIRECTION('center_axis',(-1.,0.,0.));
#140233=DIRECTION('ref_axis',(0.,0.,1.));
#140234=DIRECTION('center_axis',(1.,2.31296463463574E-15,0.));
#140235=DIRECTION('ref_axis',(-2.31296463463574E-15,1.,0.));
#140236=DIRECTION('center_axis',(0.,1.,0.));
#140237=DIRECTION('ref_axis',(0.,0.,1.));
#140238=DIRECTION('center_axis',(0.,1.,0.));
#140239=DIRECTION('ref_axis',(0.,0.,1.));
#140240=DIRECTION('center_axis',(0.,1.,0.));
#140241=DIRECTION('ref_axis',(0.,0.,1.));
#140242=DIRECTION('center_axis',(1.,0.,0.));
#140243=DIRECTION('ref_axis',(0.,0.,-1.));
#140244=DIRECTION('center_axis',(0.,-1.,0.));
#140245=DIRECTION('ref_axis',(0.,0.,-1.));
#140246=DIRECTION('center_axis',(0.,1.,0.));
#140247=DIRECTION('ref_axis',(0.,0.,1.));
#140248=DIRECTION('center_axis',(1.,0.,0.));
#140249=DIRECTION('ref_axis',(0.,0.,-1.));
#140250=DIRECTION('center_axis',(1.,0.,0.));
#140251=DIRECTION('ref_axis',(0.,0.,-1.));
#140252=DIRECTION('center_axis',(0.,0.,-1.));
#140253=DIRECTION('ref_axis',(-1.,0.,0.));
#140254=DIRECTION('center_axis',(0.,0.,1.));
#140255=DIRECTION('ref_axis',(1.,0.,0.));
#140256=DIRECTION('center_axis',(0.,0.,-1.));
#140257=DIRECTION('ref_axis',(1.,0.,0.));
#140258=DIRECTION('center_axis',(0.,0.,-1.));
#140259=DIRECTION('ref_axis',(-1.,0.,0.));
#140260=DIRECTION('center_axis',(0.,0.,1.));
#140261=DIRECTION('ref_axis',(1.,0.,0.));
#140262=DIRECTION('center_axis',(0.,0.,-1.));
#140263=DIRECTION('ref_axis',(1.,0.,0.));
#140264=DIRECTION('center_axis',(0.,0.,-1.));
#140265=DIRECTION('ref_axis',(-1.,0.,0.));
#140266=DIRECTION('center_axis',(0.,0.,1.));
#140267=DIRECTION('ref_axis',(1.,0.,0.));
#140268=DIRECTION('center_axis',(0.,0.,-1.));
#140269=DIRECTION('ref_axis',(1.,0.,0.));
#140270=DIRECTION('center_axis',(0.,0.,-1.));
#140271=DIRECTION('ref_axis',(-1.,0.,0.));
#140272=DIRECTION('center_axis',(0.,0.,1.));
#140273=DIRECTION('ref_axis',(1.,0.,0.));
#140274=DIRECTION('center_axis',(0.,0.,-1.));
#140275=DIRECTION('ref_axis',(1.,0.,0.));
#140276=DIRECTION('center_axis',(-1.,0.,0.));
#140277=DIRECTION('ref_axis',(0.,0.,1.));
#140278=DIRECTION('',(0.,0.,-1.));
#140279=DIRECTION('',(0.,1.,0.));
#140280=DIRECTION('',(0.,0.,-1.));
#140281=DIRECTION('center_axis',(0.,-1.,0.));
#140282=DIRECTION('ref_axis',(0.,0.,-1.));
#140283=DIRECTION('',(-1.,0.,0.));
#140284=DIRECTION('',(-1.,0.,0.));
#140285=DIRECTION('',(-1.,0.,0.));
#140286=DIRECTION('',(-1.,0.,0.));
#140287=DIRECTION('',(0.,0.,-1.));
#140288=DIRECTION('',(-1.,0.,0.));
#140289=DIRECTION('center_axis',(1.,0.,0.));
#140290=DIRECTION('ref_axis',(0.,0.,-1.));
#140291=DIRECTION('',(0.,-1.,0.));
#140292=DIRECTION('',(0.,0.,-1.));
#140293=DIRECTION('',(0.,-1.,0.));
#140294=DIRECTION('center_axis',(0.,1.,0.));
#140295=DIRECTION('ref_axis',(0.,0.,1.));
#140296=DIRECTION('',(1.,0.,0.));
#140297=DIRECTION('',(1.,0.,0.));
#140298=DIRECTION('',(1.,0.,0.));
#140299=DIRECTION('',(1.,0.,0.));
#140300=DIRECTION('',(1.,0.,0.));
#140301=DIRECTION('center_axis',(0.,0.,1.));
#140302=DIRECTION('ref_axis',(1.,0.,0.));
#140303=DIRECTION('',(0.,-1.,0.));
#140304=DIRECTION('center_axis',(0.,0.,1.));
#140305=DIRECTION('ref_axis',(1.,0.,0.));
#140306=DIRECTION('center_axis',(0.,0.,1.));
#140307=DIRECTION('ref_axis',(1.,0.,0.));
#140308=DIRECTION('center_axis',(0.,0.,1.));
#140309=DIRECTION('ref_axis',(1.,0.,0.));
#140310=DIRECTION('center_axis',(-1.,0.,0.));
#140311=DIRECTION('ref_axis',(0.,0.,1.));
#140312=DIRECTION('center_axis',(0.,-1.,0.));
#140313=DIRECTION('ref_axis',(0.,0.,-1.));
#140314=DIRECTION('center_axis',(0.,-1.,0.));
#140315=DIRECTION('ref_axis',(0.,0.,-1.));
#140316=DIRECTION('center_axis',(0.,-1.,0.));
#140317=DIRECTION('ref_axis',(0.,0.,-1.));
#140318=DIRECTION('center_axis',(1.,0.,0.));
#140319=DIRECTION('ref_axis',(0.,0.,-1.));
#140320=DIRECTION('center_axis',(-1.,0.,1.38777878078145E-15));
#140321=DIRECTION('ref_axis',(1.38777878078145E-15,0.,1.));
#140322=DIRECTION('center_axis',(0.,0.,1.));
#140323=DIRECTION('ref_axis',(1.,0.,0.));
#140324=DIRECTION('center_axis',(-1.,0.,0.));
#140325=DIRECTION('ref_axis',(0.,0.,1.));
#140326=DIRECTION('center_axis',(0.,0.,1.));
#140327=DIRECTION('ref_axis',(1.,0.,0.));
#140328=DIRECTION('center_axis',(0.,-1.,0.));
#140329=DIRECTION('ref_axis',(0.,0.,-1.));
#140330=DIRECTION('center_axis',(-1.,0.,0.));
#140331=DIRECTION('ref_axis',(0.,0.,1.));
#140332=DIRECTION('center_axis',(-1.,0.,0.));
#140333=DIRECTION('ref_axis',(0.,0.,1.));
#140334=DIRECTION('center_axis',(0.,1.,0.));
#140335=DIRECTION('ref_axis',(0.,0.,1.));
#140336=DIRECTION('center_axis',(0.,-1.,0.));
#140337=DIRECTION('ref_axis',(0.,0.,-1.));
#140338=DIRECTION('center_axis',(0.,0.,1.));
#140339=DIRECTION('ref_axis',(1.,0.,0.));
#140340=DIRECTION('center_axis',(0.,0.,1.));
#140341=DIRECTION('ref_axis',(1.,0.,0.));
#140342=DIRECTION('center_axis',(0.,-1.,0.));
#140343=DIRECTION('ref_axis',(0.,0.,-1.));
#140344=DIRECTION('center_axis',(-0.98587196814397,0.167500634112039,0.));
#140345=DIRECTION('ref_axis',(-0.167500634112039,-0.98587196814397,0.));
#140346=DIRECTION('center_axis',(-1.,0.,0.));
#140347=DIRECTION('ref_axis',(0.,0.,-1.));
#140348=DIRECTION('center_axis',(0.,1.,0.));
#140349=DIRECTION('ref_axis',(0.,0.,1.));
#140350=DIRECTION('center_axis',(0.,-1.,0.));
#140351=DIRECTION('ref_axis',(0.,0.,-1.));
#140352=DIRECTION('center_axis',(-1.,0.,0.));
#140353=DIRECTION('ref_axis',(0.,0.,1.));
#140354=DIRECTION('center_axis',(-1.,0.,0.));
#140355=DIRECTION('ref_axis',(0.,0.,1.));
#140356=DIRECTION('center_axis',(0.,0.,1.));
#140357=DIRECTION('ref_axis',(1.,0.,0.));
#140358=DIRECTION('center_axis',(-0.98587196814397,-0.16750063411204,1.36817219795744E-15));
#140359=DIRECTION('ref_axis',(0.16750063411204,-0.98587196814397,-7.32459110897286E-33));
#140360=DIRECTION('center_axis',(-0.98587196814397,-0.16750063411204,0.));
#140361=DIRECTION('ref_axis',(0.16750063411204,-0.98587196814397,0.));
#140362=DIRECTION('center_axis',(-1.,0.,0.));
#140363=DIRECTION('ref_axis',(0.,0.,-1.));
#140364=DIRECTION('center_axis',(0.,0.,1.));
#140365=DIRECTION('ref_axis',(1.,0.,0.));
#140366=DIRECTION('center_axis',(0.,-1.,0.));
#140367=DIRECTION('ref_axis',(0.,0.,-1.));
#140368=DIRECTION('center_axis',(1.,0.,0.));
#140369=DIRECTION('ref_axis',(0.,0.,-1.));
#140370=DIRECTION('center_axis',(-1.,0.,0.));
#140371=DIRECTION('ref_axis',(0.,0.,1.));
#140372=DIRECTION('center_axis',(0.,-1.,0.));
#140373=DIRECTION('ref_axis',(0.,0.,-1.));
#140374=DIRECTION('center_axis',(0.,-1.,0.));
#140375=DIRECTION('ref_axis',(0.,0.,-1.));
#140376=DIRECTION('center_axis',(-0.98587196814397,0.167500634112039,0.));
#140377=DIRECTION('ref_axis',(-0.167500634112039,-0.98587196814397,0.));
#140378=DIRECTION('center_axis',(0.,0.,1.));
#140379=DIRECTION('ref_axis',(1.,0.,0.));
#140380=DIRECTION('center_axis',(0.,0.,1.));
#140381=DIRECTION('ref_axis',(1.,0.,0.));
#140382=DIRECTION('',(0.,1.,0.));
#140383=DIRECTION('',(1.,0.,0.));
#140384=DIRECTION('',(0.,-1.,0.));
#140385=DIRECTION('',(-1.,0.,0.));
#140386=DIRECTION('center_axis',(-1.,0.,0.));
#140387=DIRECTION('ref_axis',(0.,0.,1.));
#140388=DIRECTION('',(0.,0.,-1.));
#140389=DIRECTION('',(0.,1.,0.));
#140390=DIRECTION('',(0.,0.,-1.));
#140391=DIRECTION('center_axis',(0.,-1.,0.));
#140392=DIRECTION('ref_axis',(0.,0.,-1.));
#140393=DIRECTION('',(0.,0.,-1.));
#140394=DIRECTION('',(-1.,0.,0.));
#140395=DIRECTION('center_axis',(1.,0.,0.));
#140396=DIRECTION('ref_axis',(0.,0.,-1.));
#140397=DIRECTION('',(0.,0.,-1.));
#140398=DIRECTION('',(0.,-1.,0.));
#140399=DIRECTION('center_axis',(0.,1.,0.));
#140400=DIRECTION('ref_axis',(0.,0.,1.));
#140401=DIRECTION('',(1.,0.,0.));
#140402=DIRECTION('center_axis',(0.,0.,1.));
#140403=DIRECTION('ref_axis',(1.,0.,0.));
#140404=DIRECTION('center_axis',(0.,1.,0.));
#140405=DIRECTION('ref_axis',(0.,0.,1.));
#140406=DIRECTION('',(-1.,0.,0.));
#140407=DIRECTION('center_axis',(0.,0.,-1.));
#140408=DIRECTION('ref_axis',(-1.,0.,0.));
#140409=DIRECTION('center_axis',(0.,-1.,0.));
#140410=DIRECTION('ref_axis',(0.,0.,-1.));
#140411=DIRECTION('',(1.,0.,0.));
#140412=DIRECTION('center_axis',(0.,0.,-1.));
#140413=DIRECTION('ref_axis',(-1.,0.,0.));
#273741=CARTESIAN_POINT('',(0.,0.,0.));
#273742=CARTESIAN_POINT('Origin',(0.,0.,0.));
#273743=CARTESIAN_POINT('',(-65.,-614.173929613455,0.));
#273744=CARTESIAN_POINT('',(65.169448912385,-614.173929613455,0.));
#273745=CARTESIAN_POINT('',(65.169448912385,-614.173929613455,0.));
#273746=CARTESIAN_POINT('',(-65.,-550.402639059603,0.));
#273747=CARTESIAN_POINT('',(-65.,-511.398533506753,0.));
#273748=CARTESIAN_POINT('',(65.169448912385,-550.402639059603,0.));
#273749=CARTESIAN_POINT('',(65.169448912385,-550.402639059603,0.));
#273750=CARTESIAN_POINT('',(65.169448912385,-511.398533506753,0.));
#273751=CARTESIAN_POINT('Origin',(0.,0.,304.));
#273752=CARTESIAN_POINT('',(49.830664447451,-620.152805159724,304.));
#273753=CARTESIAN_POINT('',(49.830664447451,-541.923394840277,304.));
#273754=CARTESIAN_POINT('',(49.830664447451,-541.923394840277,304.));
#273755=CARTESIAN_POINT('',(41.5056707885714,-532.064675158837,304.));
#273756=CARTESIAN_POINT('Origin',(39.830664447451,-541.923394840277,304.));
#273757=CARTESIAN_POINT('',(53.6812599743419,-532.064675158837,304.));
#273758=CARTESIAN_POINT('',(-53.681259974342,-532.064675158837,304.));
#273759=CARTESIAN_POINT('',(53.6812599743419,-630.011524841163,304.));
#273760=CARTESIAN_POINT('',(53.6812599743419,-532.064675158837,304.));
#273761=CARTESIAN_POINT('',(41.5056707885714,-630.011524841163,304.));
#273762=CARTESIAN_POINT('',(-53.681259974342,-630.011524841163,304.));
#273763=CARTESIAN_POINT('Origin',(39.830664447451,-620.152805159724,304.));
#273764=CARTESIAN_POINT('Origin',(-65.,-511.398533506753,25.));
#273765=CARTESIAN_POINT('',(-65.,-647.946325817004,-15.));
#273766=CARTESIAN_POINT('',(-65.,-647.946325817004,22.));
#273767=CARTESIAN_POINT('',(-65.,-647.946325817004,25.));
#273768=CARTESIAN_POINT('',(-65.,-516.398533506753,22.));
#273769=CARTESIAN_POINT('',(-65.,-516.398533506753,22.));
#273770=CARTESIAN_POINT('',(-65.,-516.398533506753,-15.));
#273771=CARTESIAN_POINT('',(-65.,-516.398533506753,25.));
#273772=CARTESIAN_POINT('',(-65.,-550.402639059603,-15.));
#273773=CARTESIAN_POINT('',(-65.,-550.402639059603,-15.));
#273774=CARTESIAN_POINT('',(-65.,-550.402639059603,-15.));
#273775=CARTESIAN_POINT('',(-65.,-614.173929613455,-15.));
#273776=CARTESIAN_POINT('',(-65.,-614.173929613455,-15.));
#273777=CARTESIAN_POINT('',(-65.,-647.946325817004,-15.));
#273778=CARTESIAN_POINT('Origin',(-65.,-652.946325817004,25.));
#273779=CARTESIAN_POINT('',(60.169448912385,-652.946325817004,-15.));
#273780=CARTESIAN_POINT('',(60.169448912385,-652.946325817004,22.));
#273781=CARTESIAN_POINT('',(60.169448912385,-652.946325817004,25.));
#273782=CARTESIAN_POINT('',(-60.,-652.946325817004,22.));
#273783=CARTESIAN_POINT('',(-60.,-652.946325817004,22.));
#273784=CARTESIAN_POINT('',(-60.,-652.946325817004,-15.));
#273785=CARTESIAN_POINT('',(-60.,-652.946325817004,25.));
#273786=CARTESIAN_POINT('',(60.169448912385,-652.946325817004,-15.));
#273787=CARTESIAN_POINT('Origin',(65.169448912385,-511.398533506753,25.));
#273788=CARTESIAN_POINT('',(65.169448912385,-516.398533506753,-15.));
#273789=CARTESIAN_POINT('',(65.169448912385,-516.398533506753,22.));
#273790=CARTESIAN_POINT('',(65.169448912385,-516.398533506753,25.));
#273791=CARTESIAN_POINT('',(65.169448912385,-647.946325817004,22.));
#273792=CARTESIAN_POINT('',(65.169448912385,-647.946325817004,22.));
#273793=CARTESIAN_POINT('',(65.169448912385,-647.946325817004,-15.));
#273794=CARTESIAN_POINT('',(65.169448912385,-647.946325817004,25.));
#273795=CARTESIAN_POINT('',(65.169448912385,-614.173929613455,-15.));
#273796=CARTESIAN_POINT('',(65.169448912385,-614.173929613455,-15.));
#273797=CARTESIAN_POINT('',(65.169448912385,-614.173929613455,-15.));
#273798=CARTESIAN_POINT('',(65.169448912385,-550.402639059603,-15.));
#273799=CARTESIAN_POINT('',(65.169448912385,-550.402639059603,-15.));
#273800=CARTESIAN_POINT('',(65.169448912385,-516.398533506753,-15.));
#273801=CARTESIAN_POINT('Origin',(-65.,-511.398533506753,25.));
#273802=CARTESIAN_POINT('',(-60.,-511.398533506753,-15.));
#273803=CARTESIAN_POINT('',(-60.,-511.398533506753,22.));
#273804=CARTESIAN_POINT('',(-60.,-511.398533506753,25.));
#273805=CARTESIAN_POINT('',(60.169448912385,-511.398533506753,22.));
#273806=CARTESIAN_POINT('',(60.169448912385,-511.398533506753,22.));
#273807=CARTESIAN_POINT('',(60.169448912385,-511.398533506753,-15.));
#273808=CARTESIAN_POINT('',(60.169448912385,-511.398533506753,25.));
#273809=CARTESIAN_POINT('',(-60.,-511.398533506753,-15.));
#273810=CARTESIAN_POINT('Origin',(0.,0.,25.));
#273811=CARTESIAN_POINT('',(62.169448912385,-647.946325817004,25.));
#273812=CARTESIAN_POINT('',(62.169448912385,-516.398533506753,25.));
#273813=CARTESIAN_POINT('',(62.169448912385,-516.398533506753,25.));
#273814=CARTESIAN_POINT('',(60.169448912385,-514.398533506753,25.));
#273815=CARTESIAN_POINT('Origin',(60.169448912385,-516.398533506753,25.));
#273816=CARTESIAN_POINT('',(-60.,-514.398533506753,25.));
#273817=CARTESIAN_POINT('',(-60.,-514.398533506753,25.));
#273818=CARTESIAN_POINT('',(-62.,-516.398533506753,25.));
#273819=CARTESIAN_POINT('Origin',(-60.,-516.398533506753,25.));
#273820=CARTESIAN_POINT('',(-62.,-647.946325817004,25.));
#273821=CARTESIAN_POINT('',(-62.,-647.946325817004,25.));
#273822=CARTESIAN_POINT('',(-60.,-649.946325817004,25.));
#273823=CARTESIAN_POINT('Origin',(-60.,-647.946325817004,25.));
#273824=CARTESIAN_POINT('',(60.169448912385,-649.946325817004,25.));
#273825=CARTESIAN_POINT('',(60.169448912385,-649.946325817004,25.));
#273826=CARTESIAN_POINT('Origin',(60.169448912385,-647.946325817004,25.));
#273827=CARTESIAN_POINT('',(-39.830664447451,-531.923394840277,25.));
#273828=CARTESIAN_POINT('',(39.830664447451,-531.923394840277,25.));
#273829=CARTESIAN_POINT('',(0.,-531.923394840277,25.));
#273830=CARTESIAN_POINT('',(49.830664447451,-541.923394840277,25.));
#273831=CARTESIAN_POINT('Origin',(39.830664447451,-541.923394840277,25.));
#273832=CARTESIAN_POINT('',(49.830664447451,-620.152805159724,25.));
#273833=CARTESIAN_POINT('',(49.830664447451,0.,25.));
#273834=CARTESIAN_POINT('',(39.830664447451,-630.152805159724,25.));
#273835=CARTESIAN_POINT('Origin',(39.830664447451,-620.152805159724,25.));
#273836=CARTESIAN_POINT('',(-39.830664447451,-630.152805159724,25.));
#273837=CARTESIAN_POINT('',(0.,-630.152805159724,25.));
#273838=CARTESIAN_POINT('',(-49.830664447451,-620.152805159724,25.));
#273839=CARTESIAN_POINT('Origin',(-39.830664447451,-620.152805159724,25.));
#273840=CARTESIAN_POINT('',(-49.830664447451,-541.923394840277,25.));
#273841=CARTESIAN_POINT('',(-49.830664447451,0.,25.));
#273842=CARTESIAN_POINT('Origin',(-39.830664447451,-541.923394840277,25.));
#273843=CARTESIAN_POINT('Origin',(44.830664447451,-536.923394840277,304.));
#273844=CARTESIAN_POINT('',(44.830664447451,-620.152805159724,299.));
#273845=CARTESIAN_POINT('',(44.830664447451,-620.152805159724,30.));
#273846=CARTESIAN_POINT('',(44.830664447451,-620.152805159724,304.));
#273847=CARTESIAN_POINT('',(44.830664447451,-541.923394840277,30.));
#273848=CARTESIAN_POINT('',(44.830664447451,-536.923394840277,30.));
#273849=CARTESIAN_POINT('',(44.830664447451,-541.923394840277,299.));
#273850=CARTESIAN_POINT('',(44.830664447451,-541.923394840277,304.));
#273851=CARTESIAN_POINT('',(44.830664447451,-620.152805159724,299.));
#273852=CARTESIAN_POINT('Origin',(-44.830664447451,-536.923394840277,304.));
#273853=CARTESIAN_POINT('',(-39.830664447451,-536.923394840277,30.));
#273854=CARTESIAN_POINT('',(-39.830664447451,-536.923394840277,299.001996411407));
#273855=CARTESIAN_POINT('',(-39.830664447451,-536.923394840277,304.));
#273856=CARTESIAN_POINT('',(39.830664447451,-536.923394840277,299.001996411407));
#273857=CARTESIAN_POINT('',(-44.830664447451,-536.923394840277,299.001996411407));
#273858=CARTESIAN_POINT('',(39.830664447451,-536.923394840277,30.));
#273859=CARTESIAN_POINT('',(39.830664447451,-536.923394840277,304.));
#273860=CARTESIAN_POINT('',(-44.830664447451,-536.923394840277,30.));
#273861=CARTESIAN_POINT('Origin',(-44.830664447451,-536.923394840277,304.));
#273862=CARTESIAN_POINT('',(-44.830664447451,-541.923394840277,299.));
#273863=CARTESIAN_POINT('',(-44.830664447451,-541.923394840277,30.));
#273864=CARTESIAN_POINT('',(-44.830664447451,-541.923394840277,304.));
#273865=CARTESIAN_POINT('',(-44.830664447451,-620.152805159724,30.));
#273866=CARTESIAN_POINT('',(-44.830664447451,-536.923394840277,30.));
#273867=CARTESIAN_POINT('',(-44.830664447451,-620.152805159724,299.));
#273868=CARTESIAN_POINT('',(-44.830664447451,-620.152805159724,304.));
#273869=CARTESIAN_POINT('',(-44.830664447451,-541.923394840277,299.));
#273870=CARTESIAN_POINT('Origin',(-44.830664447451,-625.152805159724,304.));
#273871=CARTESIAN_POINT('',(-39.830664447451,-625.152805159724,299.001996411407));
#273872=CARTESIAN_POINT('',(-39.830664447451,-625.152805159724,30.));
#273873=CARTESIAN_POINT('',(-39.830664447451,-625.152805159724,304.));
#273874=CARTESIAN_POINT('',(39.830664447451,-625.152805159724,30.));
#273875=CARTESIAN_POINT('',(-44.830664447451,-625.152805159724,30.));
#273876=CARTESIAN_POINT('',(39.830664447451,-625.152805159724,299.001996411407));
#273877=CARTESIAN_POINT('',(39.830664447451,-625.152805159724,304.));
#273878=CARTESIAN_POINT('',(-44.830664447451,-625.152805159724,299.001996411407));
#273879=CARTESIAN_POINT('Origin',(-60.,-516.398533506753,25.));
#273880=CARTESIAN_POINT('Origin',(-60.,-516.398533506753,22.));
#273881=CARTESIAN_POINT('Origin',(-60.,-516.398533506753,-15.));
#273882=CARTESIAN_POINT('Origin',(60.169448912385,-647.946325817004,25.));
#273883=CARTESIAN_POINT('Origin',(60.169448912385,-647.946325817004,22.));
#273884=CARTESIAN_POINT('Origin',(60.169448912385,-647.946325817004,-15.));
#273885=CARTESIAN_POINT('Origin',(-60.,-647.946325817004,25.));
#273886=CARTESIAN_POINT('Origin',(-60.,-647.946325817004,22.));
#273887=CARTESIAN_POINT('Origin',(-60.,-647.946325817004,-15.));
#273888=CARTESIAN_POINT('Origin',(60.169448912385,-516.398533506753,25.));
#273889=CARTESIAN_POINT('Origin',(60.169448912385,-516.398533506753,22.));
#273890=CARTESIAN_POINT('Origin',(60.169448912385,-516.398533506753,-15.));
#273891=CARTESIAN_POINT('Ctrl Pts',(-65.,-647.946325817004,22.));
#273892=CARTESIAN_POINT('Ctrl Pts',(-65.,-652.946325817004,22.));
#273893=CARTESIAN_POINT('Ctrl Pts',(-60.,-652.946325817004,22.));
#273894=CARTESIAN_POINT('Ctrl Pts',(-65.,-647.946325817004,25.));
#273895=CARTESIAN_POINT('Ctrl Pts',(-65.,-652.946325817004,25.));
#273896=CARTESIAN_POINT('Ctrl Pts',(-60.,-652.946325817004,25.));
#273897=CARTESIAN_POINT('Ctrl Pts',(-62.,-647.946325817004,25.));
#273898=CARTESIAN_POINT('Ctrl Pts',(-62.,-649.946325817004,25.));
#273899=CARTESIAN_POINT('Ctrl Pts',(-60.,-649.946325817004,25.));
#273900=CARTESIAN_POINT('Origin',(-62.,-647.946325817004,22.));
#273901=CARTESIAN_POINT('Origin',(-60.,-649.946325817004,22.));
#273902=CARTESIAN_POINT('Origin',(0.,-649.946325817004,22.));
#273903=CARTESIAN_POINT('Origin',(60.169448912385,-649.946325817004,22.));
#273904=CARTESIAN_POINT('Origin',(-62.,0.,22.));
#273905=CARTESIAN_POINT('Origin',(-62.,-516.398533506753,22.));
#273906=CARTESIAN_POINT('Ctrl Pts',(60.169448912385,-652.946325817004,22.));
#273907=CARTESIAN_POINT('Ctrl Pts',(65.169448912385,-652.946325817004,22.));
#273908=CARTESIAN_POINT('Ctrl Pts',(65.169448912385,-647.946325817004,22.));
#273909=CARTESIAN_POINT('Ctrl Pts',(60.169448912385,-652.946325817004,25.));
#273910=CARTESIAN_POINT('Ctrl Pts',(65.169448912385,-652.946325817004,25.));
#273911=CARTESIAN_POINT('Ctrl Pts',(65.169448912385,-647.946325817004,25.));
#273912=CARTESIAN_POINT('Ctrl Pts',(60.169448912385,-649.946325817004,25.));
#273913=CARTESIAN_POINT('Ctrl Pts',(62.169448912385,-649.946325817004,25.));
#273914=CARTESIAN_POINT('Ctrl Pts',(62.169448912385,-647.946325817004,25.));
#273915=CARTESIAN_POINT('Origin',(62.169448912385,-647.946325817004,22.));
#273916=CARTESIAN_POINT('Ctrl Pts',(-60.,-511.398533506753,22.));
#273917=CARTESIAN_POINT('Ctrl Pts',(-65.,-511.398533506753,22.));
#273918=CARTESIAN_POINT('Ctrl Pts',(-65.,-516.398533506753,22.));
#273919=CARTESIAN_POINT('Ctrl Pts',(-60.,-511.398533506753,25.));
#273920=CARTESIAN_POINT('Ctrl Pts',(-65.,-511.398533506753,25.));
#273921=CARTESIAN_POINT('Ctrl Pts',(-65.,-516.398533506753,25.));
#273922=CARTESIAN_POINT('Ctrl Pts',(-60.,-514.398533506753,25.));
#273923=CARTESIAN_POINT('Ctrl Pts',(-62.,-514.398533506753,25.));
#273924=CARTESIAN_POINT('Ctrl Pts',(-62.,-516.398533506753,25.));
#273925=CARTESIAN_POINT('Origin',(-60.,-514.398533506753,22.));
#273926=CARTESIAN_POINT('Origin',(62.169448912385,0.,22.));
#273927=CARTESIAN_POINT('Origin',(62.169448912385,-516.398533506753,22.));
#273928=CARTESIAN_POINT('Origin',(0.,-514.398533506753,22.));
#273929=CARTESIAN_POINT('Origin',(60.169448912385,-514.398533506753,22.));
#273930=CARTESIAN_POINT('Ctrl Pts',(65.169448912385,-516.398533506753,22.));
#273931=CARTESIAN_POINT('Ctrl Pts',(65.169448912385,-511.398533506753,22.));
#273932=CARTESIAN_POINT('Ctrl Pts',(60.169448912385,-511.398533506753,22.));
#273933=CARTESIAN_POINT('Ctrl Pts',(65.169448912385,-516.398533506753,25.));
#273934=CARTESIAN_POINT('Ctrl Pts',(65.169448912385,-511.398533506753,25.));
#273935=CARTESIAN_POINT('Ctrl Pts',(60.169448912385,-511.398533506753,25.));
#273936=CARTESIAN_POINT('Ctrl Pts',(62.169448912385,-516.398533506753,25.));
#273937=CARTESIAN_POINT('Ctrl Pts',(62.169448912385,-514.398533506753,25.));
#273938=CARTESIAN_POINT('Ctrl Pts',(60.169448912385,-514.398533506753,25.));
#273939=CARTESIAN_POINT('Origin',(39.830664447451,-620.152805159724,304.));
#273940=CARTESIAN_POINT('Origin',(39.830664447451,-620.152805159724,30.));
#273941=CARTESIAN_POINT('',(40.6681676180112,-625.082165000443,299.));
#273942=CARTESIAN_POINT('Origin',(39.830664447451,-620.152805159724,299.));
#273943=CARTESIAN_POINT('Ctrl Pts',(40.6681676180112,-625.082165000443,
299.));
#273944=CARTESIAN_POINT('Ctrl Pts',(40.5568123862982,-625.101084365763,
299.));
#273945=CARTESIAN_POINT('Ctrl Pts',(40.4451315445969,-625.116181235656,
299.000322224733));
#273946=CARTESIAN_POINT('Ctrl Pts',(40.3331319375785,-625.127493735038,
299.000707767503));
#273947=CARTESIAN_POINT('Ctrl Pts',(40.221073548286,-625.138812171713,299.001093512622));
#273948=CARTESIAN_POINT('Ctrl Pts',(40.1086953597897,-625.146342339687,
299.001542642259));
#273949=CARTESIAN_POINT('Ctrl Pts',(39.9959972959025,-625.150070917038,
299.001795841848));
#273950=CARTESIAN_POINT('Ctrl Pts',(39.9409626133207,-625.151891720908,
299.001919488684));
#273951=CARTESIAN_POINT('Ctrl Pts',(39.8858516096048,-625.152805159724,
299.001996411407));
#273952=CARTESIAN_POINT('Ctrl Pts',(39.830664447451,-625.152805159724,299.001996411407));
#273953=CARTESIAN_POINT('Origin',(-39.830664447451,-620.152805159724,304.));
#273954=CARTESIAN_POINT('Origin',(-39.830664447451,-620.152805159724,30.));
#273955=CARTESIAN_POINT('',(-40.6681676180112,-625.082165000443,299.));
#273956=CARTESIAN_POINT('Ctrl Pts',(-39.830664447451,-625.152805159724,
299.001996411407));
#273957=CARTESIAN_POINT('Ctrl Pts',(-39.9432259736778,-625.152805159724,
299.001996411407));
#273958=CARTESIAN_POINT('Ctrl Pts',(-40.055467122883,-625.149008478778,
299.001676420839));
#273959=CARTESIAN_POINT('Ctrl Pts',(-40.1673902027881,-625.141453851072,
299.001292658354));
#273960=CARTESIAN_POINT('Ctrl Pts',(-40.2793727095621,-625.133895212148,
299.000908692105));
#273961=CARTESIAN_POINT('Ctrl Pts',(-40.3910375070763,-625.122574592185,
299.000460886201));
#273962=CARTESIAN_POINT('Ctrl Pts',(-40.5023851435054,-625.107478842873,
299.000205867636));
#273963=CARTESIAN_POINT('Ctrl Pts',(-40.5577247055267,-625.09997628438,
299.000079123898));
#273964=CARTESIAN_POINT('Ctrl Pts',(-40.6129858337698,-625.091540440815,
299.));
#273965=CARTESIAN_POINT('Ctrl Pts',(-40.6681676180113,-625.082165000443,
299.));
#273966=CARTESIAN_POINT('Origin',(-39.830664447451,-620.152805159724,299.));
#273967=CARTESIAN_POINT('Origin',(39.830664447451,-541.923394840277,304.));
#273968=CARTESIAN_POINT('Origin',(39.830664447451,-541.923394840277,30.));
#273969=CARTESIAN_POINT('',(40.6681676180112,-536.994034999557,299.));
#273970=CARTESIAN_POINT('Ctrl Pts',(39.830664447451,-536.923394840277,299.001996411407));
#273971=CARTESIAN_POINT('Ctrl Pts',(39.9432259736786,-536.923394840277,
299.001996411407));
#273972=CARTESIAN_POINT('Ctrl Pts',(40.0554671228846,-536.927191521222,
299.001676420839));
#273973=CARTESIAN_POINT('Ctrl Pts',(40.1673902027906,-536.934746148928,
299.001292658354));
#273974=CARTESIAN_POINT('Ctrl Pts',(40.279372709565,-536.942304787853,299.000908692105));
#273975=CARTESIAN_POINT('Ctrl Pts',(40.3910375070795,-536.953625407815,
299.000460886201));
#273976=CARTESIAN_POINT('Ctrl Pts',(40.502385143509,-536.968721157128,299.000205867636));
#273977=CARTESIAN_POINT('Ctrl Pts',(40.557724705529,-536.97622371562,299.000079123898));
#273978=CARTESIAN_POINT('Ctrl Pts',(40.6129858337709,-536.984659559185,
299.));
#273979=CARTESIAN_POINT('Ctrl Pts',(40.6681676180112,-536.994034999557,
299.));
#273980=CARTESIAN_POINT('Origin',(39.830664447451,-541.923394840277,299.));
#273981=CARTESIAN_POINT('Origin',(-39.830664447451,-541.923394840277,304.));
#273982=CARTESIAN_POINT('Origin',(-39.830664447451,-541.923394840277,30.));
#273983=CARTESIAN_POINT('',(-40.6681676180112,-536.994034999557,299.));
#273984=CARTESIAN_POINT('Origin',(-39.830664447451,-541.923394840277,299.));
#273985=CARTESIAN_POINT('Ctrl Pts',(-40.6681676180112,-536.994034999557,
299.));
#273986=CARTESIAN_POINT('Ctrl Pts',(-40.5568123862973,-536.975115634237,
299.));
#273987=CARTESIAN_POINT('Ctrl Pts',(-40.4451315445951,-536.960018764344,
299.000322224733));
#273988=CARTESIAN_POINT('Ctrl Pts',(-40.3331319375757,-536.948706264962,
299.000707767503));
#273989=CARTESIAN_POINT('Ctrl Pts',(-40.221073548282,-536.937387828287,
299.001093512622));
#273990=CARTESIAN_POINT('Ctrl Pts',(-40.1086953597845,-536.929857660313,
299.001542642259));
#273991=CARTESIAN_POINT('Ctrl Pts',(-39.9959972958961,-536.926129082962,
299.001795841848));
#273992=CARTESIAN_POINT('Ctrl Pts',(-39.9409626133164,-536.924308279092,
299.001919488684));
#273993=CARTESIAN_POINT('Ctrl Pts',(-39.8858516096027,-536.923394840277,
299.001996411407));
#273994=CARTESIAN_POINT('Ctrl Pts',(-39.830664447451,-536.923394840277,
299.001996411407));
#273995=CARTESIAN_POINT('Origin',(53.6812599743419,-532.064675158837,346.));
#273996=CARTESIAN_POINT('',(53.6812599743419,-532.064675158837,346.));
#273997=CARTESIAN_POINT('',(53.6812599743419,-532.064675158837,346.));
#273998=CARTESIAN_POINT('',(53.6812599743419,-630.011524841163,346.));
#273999=CARTESIAN_POINT('',(53.6812599743419,-532.064675158837,346.));
#274000=CARTESIAN_POINT('',(53.6812599743419,-630.011524841163,346.));
#274001=CARTESIAN_POINT('Origin',(-53.681259974342,-532.064675158837,346.));
#274002=CARTESIAN_POINT('',(39.830664447451,-532.064675158837,304.));
#274003=CARTESIAN_POINT('',(-53.681259974342,-532.064675158837,304.));
#274004=CARTESIAN_POINT('',(-39.830664447451,-532.064675158837,304.));
#274005=CARTESIAN_POINT('',(-53.681259974342,-532.064675158837,304.));
#274006=CARTESIAN_POINT('',(-41.5056707885714,-532.064675158837,304.));
#274007=CARTESIAN_POINT('',(-53.681259974342,-532.064675158837,304.));
#274008=CARTESIAN_POINT('',(-53.681259974342,-532.064675158837,304.));
#274009=CARTESIAN_POINT('',(-53.681259974342,-532.064675158837,304.));
#274010=CARTESIAN_POINT('',(-53.681259974342,-532.064675158837,346.));
#274011=CARTESIAN_POINT('',(-53.681259974342,-532.064675158837,346.));
#274012=CARTESIAN_POINT('',(-53.681259974342,-532.064675158837,346.));
#274013=CARTESIAN_POINT('Origin',(-53.681259974342,-532.064675158837,346.));
#274014=CARTESIAN_POINT('',(-53.681259974342,-630.011524841163,304.));
#274015=CARTESIAN_POINT('',(-53.681259974342,-532.064675158837,304.));
#274016=CARTESIAN_POINT('',(-53.681259974342,-630.011524841163,346.));
#274017=CARTESIAN_POINT('',(-53.681259974342,-630.011524841163,346.));
#274018=CARTESIAN_POINT('',(-53.681259974342,-532.064675158837,346.));
#274019=CARTESIAN_POINT('Origin',(-53.681259974342,-630.011524841163,346.));
#274020=CARTESIAN_POINT('',(-41.5056707885714,-630.011524841163,304.));
#274021=CARTESIAN_POINT('',(-53.681259974342,-630.011524841163,304.));
#274022=CARTESIAN_POINT('',(-39.830664447451,-630.011524841163,304.));
#274023=CARTESIAN_POINT('',(-53.681259974342,-630.011524841163,304.));
#274024=CARTESIAN_POINT('',(39.830664447451,-630.011524841163,304.));
#274025=CARTESIAN_POINT('',(-53.681259974342,-630.011524841163,304.));
#274026=CARTESIAN_POINT('',(-53.681259974342,-630.011524841163,304.));
#274027=CARTESIAN_POINT('',(-53.681259974342,-630.011524841163,346.));
#274028=CARTESIAN_POINT('Origin',(0.,0.,304.));
#274029=CARTESIAN_POINT('',(-49.830664447451,-541.923394840277,304.));
#274030=CARTESIAN_POINT('',(-49.830664447451,-620.152805159724,304.));
#274031=CARTESIAN_POINT('',(-49.830664447451,-620.152805159724,304.));
#274032=CARTESIAN_POINT('Origin',(-39.830664447451,-620.152805159724,304.));
#274033=CARTESIAN_POINT('Origin',(-39.830664447451,-541.923394840277,304.));
#274034=CARTESIAN_POINT('Origin',(-39.830664447451,-620.152805159724,30.));
#274035=CARTESIAN_POINT('Origin',(-39.830664447451,-630.152805159724,30.));
#274036=CARTESIAN_POINT('Origin',(-49.830664447451,-620.152805159724,30.));
#274037=CARTESIAN_POINT('Origin',(-49.830664447451,-536.923394840277,30.));
#274038=CARTESIAN_POINT('Origin',(-49.830664447451,-541.923394840277,30.));
#274039=CARTESIAN_POINT('Origin',(-44.830664447451,-630.152805159724,30.));
#274040=CARTESIAN_POINT('Origin',(39.830664447451,-630.152805159724,30.));
#274041=CARTESIAN_POINT('Origin',(-39.830664447451,-541.923394840277,30.));
#274042=CARTESIAN_POINT('Origin',(-39.830664447451,-531.923394840277,30.));
#274043=CARTESIAN_POINT('Origin',(39.830664447451,-620.152805159724,30.));
#274044=CARTESIAN_POINT('Origin',(49.830664447451,-620.152805159724,30.));
#274045=CARTESIAN_POINT('Origin',(-44.830664447451,-531.923394840277,30.));
#274046=CARTESIAN_POINT('Origin',(39.830664447451,-531.923394840277,30.));
#274047=CARTESIAN_POINT('Origin',(49.830664447451,-536.923394840277,30.));
#274048=CARTESIAN_POINT('Origin',(49.830664447451,-541.923394840277,30.));
#274049=CARTESIAN_POINT('Origin',(39.830664447451,-541.923394840277,30.));
#274050=CARTESIAN_POINT('Origin',(-39.830664447451,-620.152805159724,299.));
#274051=CARTESIAN_POINT('Origin',(-49.830664447451,-620.152805159724,299.));
#274052=CARTESIAN_POINT('Origin',(-41.5056707885714,-630.011524841163,299.));
#274053=CARTESIAN_POINT('Ctrl Pts',(-39.830664447451,-625.152805159724,
299.001996411407));
#274054=CARTESIAN_POINT('Ctrl Pts',(-39.830664447451,-625.152805159724,
303.862656868443));
#274055=CARTESIAN_POINT('Ctrl Pts',(-39.830664447451,-630.011524841163,
304.));
#274056=CARTESIAN_POINT('Ctrl Pts',(-40.1099566802916,-625.152805159724,
299.001996411454));
#274057=CARTESIAN_POINT('Ctrl Pts',(-40.1174997460946,-625.152805159662,
303.862656868474));
#274058=CARTESIAN_POINT('Ctrl Pts',(-40.3892847158792,-630.011524841163,
304.));
#274059=CARTESIAN_POINT('Ctrl Pts',(-40.389168630662,-625.129567207634,
299.000000001807));
#274060=CARTESIAN_POINT('Ctrl Pts',(-40.4072487687408,-625.126495377405,
303.907395550511));
#274061=CARTESIAN_POINT('Ctrl Pts',(-40.9476251437622,-630.011524841163,
304.));
#274062=CARTESIAN_POINT('Ctrl Pts',(-40.6681676180112,-625.082165000443,
299.));
#274063=CARTESIAN_POINT('Ctrl Pts',(-40.6681676180112,-625.082165000443,
304.));
#274064=CARTESIAN_POINT('Ctrl Pts',(-41.5056707885714,-630.011524841163,
304.));
#274065=CARTESIAN_POINT('Origin',(-39.830664447451,-630.152805159724,299.001996411407));
#274066=CARTESIAN_POINT('Origin',(-49.830664447451,0.,299.));
#274067=CARTESIAN_POINT('Origin',(-49.830664447451,-541.923394840277,299.));
#274068=CARTESIAN_POINT('Origin',(0.,-630.152805159724,299.001996411407));
#274069=CARTESIAN_POINT('Origin',(39.830664447451,-630.152805159724,299.001996411407));
#274070=CARTESIAN_POINT('Origin',(-39.830664447451,-541.923394840277,299.));
#274071=CARTESIAN_POINT('Origin',(-41.5056707885714,-532.064675158837,299.));
#274072=CARTESIAN_POINT('Ctrl Pts',(39.830664447451,-630.011524841163,304.));
#274073=CARTESIAN_POINT('Ctrl Pts',(39.830664447451,-625.152805159724,303.862656868443));
#274074=CARTESIAN_POINT('Ctrl Pts',(39.830664447451,-625.152805159724,299.001996411407));
#274075=CARTESIAN_POINT('Ctrl Pts',(40.3892847158792,-630.011524841165,
304.));
#274076=CARTESIAN_POINT('Ctrl Pts',(40.1174997461169,-625.152805159662,
303.862656868536));
#274077=CARTESIAN_POINT('Ctrl Pts',(40.1099566802917,-625.152805159724,
299.001996411454));
#274078=CARTESIAN_POINT('Ctrl Pts',(40.9476251437621,-630.011524841163,
304.));
#274079=CARTESIAN_POINT('Ctrl Pts',(40.4072487687113,-625.126495377409,
303.907395550502));
#274080=CARTESIAN_POINT('Ctrl Pts',(40.3891686306619,-625.129567207634,
299.000000001807));
#274081=CARTESIAN_POINT('Ctrl Pts',(41.5056707885714,-630.011524841163,
304.));
#274082=CARTESIAN_POINT('Ctrl Pts',(40.6681676180112,-625.082165000443,
304.));
#274083=CARTESIAN_POINT('Ctrl Pts',(40.6681676180112,-625.082165000443,
299.));
#274084=CARTESIAN_POINT('Origin',(41.5056707885714,-630.011524841163,299.));
#274085=CARTESIAN_POINT('Ctrl Pts',(-39.830664447451,-532.064675158837,
304.));
#274086=CARTESIAN_POINT('Ctrl Pts',(-39.830664447451,-536.923394840277,
303.862656868443));
#274087=CARTESIAN_POINT('Ctrl Pts',(-39.830664447451,-536.923394840277,
299.001996411407));
#274088=CARTESIAN_POINT('Ctrl Pts',(-40.3892847158792,-532.064675158837,
304.));
#274089=CARTESIAN_POINT('Ctrl Pts',(-40.117499746096,-536.923394840339,
303.862656868474));
#274090=CARTESIAN_POINT('Ctrl Pts',(-40.1099566802916,-536.923394840277,
299.001996411454));
#274091=CARTESIAN_POINT('Ctrl Pts',(-40.9476251437622,-532.064675158837,
304.));
#274092=CARTESIAN_POINT('Ctrl Pts',(-40.4072487687389,-536.949704622596,
303.907395550513));
#274093=CARTESIAN_POINT('Ctrl Pts',(-40.389168630662,-536.946632792366,
299.000000001807));
#274094=CARTESIAN_POINT('Ctrl Pts',(-41.5056707885714,-532.064675158837,
304.));
#274095=CARTESIAN_POINT('Ctrl Pts',(-40.6681676180112,-536.994034999557,
304.));
#274096=CARTESIAN_POINT('Ctrl Pts',(-40.6681676180112,-536.994034999557,
299.));
#274097=CARTESIAN_POINT('Origin',(-39.830664447451,-531.923394840277,299.001996411407));
#274098=CARTESIAN_POINT('Origin',(39.830664447451,-620.152805159724,299.));
#274099=CARTESIAN_POINT('Origin',(49.830664447451,-620.152805159724,299.));
#274100=CARTESIAN_POINT('Origin',(0.,-531.923394840277,299.001996411407));
#274101=CARTESIAN_POINT('Origin',(39.830664447451,-531.923394840277,299.001996411407));
#274102=CARTESIAN_POINT('Origin',(49.830664447451,0.,299.));
#274103=CARTESIAN_POINT('Origin',(49.830664447451,-541.923394840277,299.));
#274104=CARTESIAN_POINT('Ctrl Pts',(39.830664447451,-536.923394840277,299.001996411407));
#274105=CARTESIAN_POINT('Ctrl Pts',(39.830664447451,-536.923394840277,303.862656868443));
#274106=CARTESIAN_POINT('Ctrl Pts',(39.830664447451,-532.064675158837,304.));
#274107=CARTESIAN_POINT('Ctrl Pts',(40.1099566802915,-536.923394840277,
299.001996411454));
#274108=CARTESIAN_POINT('Ctrl Pts',(40.117499746096,-536.923394840339,303.862656868474));
#274109=CARTESIAN_POINT('Ctrl Pts',(40.3892847158792,-532.064675158837,
304.));
#274110=CARTESIAN_POINT('Ctrl Pts',(40.389168630662,-536.946632792366,299.000000001807));
#274111=CARTESIAN_POINT('Ctrl Pts',(40.4072487687388,-536.949704622596,
303.907395550513));
#274112=CARTESIAN_POINT('Ctrl Pts',(40.9476251437621,-532.064675158837,
304.));
#274113=CARTESIAN_POINT('Ctrl Pts',(40.6681676180112,-536.994034999557,
299.));
#274114=CARTESIAN_POINT('Ctrl Pts',(40.6681676180112,-536.994034999557,
304.));
#274115=CARTESIAN_POINT('Ctrl Pts',(41.5056707885714,-532.064675158837,
304.));
#274116=CARTESIAN_POINT('Origin',(41.5056707885714,-532.064675158837,299.));
#274117=CARTESIAN_POINT('Origin',(39.830664447451,-541.923394840277,299.));
#274118=CARTESIAN_POINT('Origin',(0.,0.,346.));
#274119=CARTESIAN_POINT('',(60.9525837346152,-637.028433422628,346.));
#274120=CARTESIAN_POINT('',(60.9525837346152,-525.047766577373,346.));
#274121=CARTESIAN_POINT('',(60.9525837346152,-525.047766577373,346.));
#274122=CARTESIAN_POINT('',(-60.9525837346153,-637.028433422628,346.));
#274123=CARTESIAN_POINT('',(-60.9525837346153,-637.028433422628,346.));
#274124=CARTESIAN_POINT('',(-60.9525837346153,-525.047766577373,346.));
#274125=CARTESIAN_POINT('',(-60.9525837346153,-525.047766577373,346.));
#274126=CARTESIAN_POINT('',(-60.9525837346153,-525.047766577373,346.));
#274127=CARTESIAN_POINT('Origin',(60.9525837346152,-525.047766577373,356.));
#274128=CARTESIAN_POINT('',(60.9525837346152,-525.047766577373,356.));
#274129=CARTESIAN_POINT('',(60.9525837346152,-525.047766577373,356.));
#274130=CARTESIAN_POINT('',(60.9525837346152,-637.028433422628,356.));
#274131=CARTESIAN_POINT('',(60.9525837346152,-525.047766577373,356.));
#274132=CARTESIAN_POINT('',(60.9525837346152,-637.028433422628,356.));
#274133=CARTESIAN_POINT('Origin',(-60.9525837346153,-525.047766577373,356.));
#274134=CARTESIAN_POINT('',(-60.9525837346153,-525.047766577373,356.));
#274135=CARTESIAN_POINT('',(-60.9525837346153,-525.047766577373,356.));
#274136=CARTESIAN_POINT('',(-60.9525837346153,-525.047766577373,356.));
#274137=CARTESIAN_POINT('Origin',(-60.9525837346153,-525.047766577373,356.));
#274138=CARTESIAN_POINT('',(-60.9525837346153,-637.028433422628,356.));
#274139=CARTESIAN_POINT('',(-60.9525837346153,-637.028433422628,356.));
#274140=CARTESIAN_POINT('',(-60.9525837346153,-525.047766577373,356.));
#274141=CARTESIAN_POINT('Origin',(-60.9525837346153,-637.028433422628,356.));
#274142=CARTESIAN_POINT('',(-60.9525837346153,-637.028433422628,356.));
#274143=CARTESIAN_POINT('Origin',(0.,0.,356.));
#274144=CARTESIAN_POINT('Origin',(65.169448912385,-550.402639059603,-15.));
#274145=CARTESIAN_POINT('',(65.169448912385,-550.402639059603,-15.));
#274146=CARTESIAN_POINT('Origin',(-60.,-516.398533506753,-15.));
#274147=CARTESIAN_POINT('Origin',(65.169448912385,-614.173929613455,-15.));
#274148=CARTESIAN_POINT('',(65.169448912385,-614.173929613455,-15.));
#274149=CARTESIAN_POINT('Origin',(-60.,-647.946325817004,-15.));
#276452=UNCERTAINTY_MEASURE_WITH_UNIT(LENGTH_MEASURE(0.01),#276463,
'DISTANCE_ACCURACY_VALUE',
'Maximum model space distance between geometric entities at asserted c
onnectivities');
#276454=UNCERTAINTY_MEASURE_WITH_UNIT(LENGTH_MEASURE(0.01),#276463,
'DISTANCE_ACCURACY_VALUE',
'Maximum model space distance between geometric entities at asserted c
onnectivities');
#276460=(
GEOMETRIC_REPRESENTATION_CONTEXT(3)
GLOBAL_UNCERTAINTY_ASSIGNED_CONTEXT((#276452))
GLOBAL_UNIT_ASSIGNED_CONTEXT((#276463,#276465,#276466))
REPRESENTATION_CONTEXT('','3D')
);
#276462=(
GEOMETRIC_REPRESENTATION_CONTEXT(3)
GLOBAL_UNCERTAINTY_ASSIGNED_CONTEXT((#276454))
GLOBAL_UNIT_ASSIGNED_CONTEXT((#276463,#276465,#276466))
REPRESENTATION_CONTEXT('','3D')
);
#276463=(
LENGTH_UNIT()
NAMED_UNIT(*)
SI_UNIT(.MILLI.,.METRE.)
);
#276465=(
NAMED_UNIT(*)
PLANE_ANGLE_UNIT()
SI_UNIT($,.RADIAN.)
);
#276466=(
NAMED_UNIT(*)
SI_UNIT($,.STERADIAN.)
SOLID_ANGLE_UNIT()
);
#276472=SHAPE_DEFINITION_REPRESENTATION(#276479,#276492);
#276479=PRODUCT_DEFINITION_SHAPE('',$,#276500);
#276492=SHAPE_REPRESENTATION('',(#110875),#276460);
#276494=PRODUCT_DEFINITION_CONTEXT('part definition',#276517,'design');
#276500=PRODUCT_DEFINITION('hopper connector arm',
'hopper connector arm',#276507,#276494);
#276507=PRODUCT_DEFINITION_FORMATION('',$,#276524);
#276517=APPLICATION_CONTEXT(
'Core Data for Automotive Mechanical Design Process');
#276518=PRODUCT_CONTEXT('part definition',#276517,'mechanical');
#276524=PRODUCT('hopper connector arm','hopper connector arm',$,(#276518));
#276527=PRESENTATION_STYLE_ASSIGNMENT((#276532));
#276532=SURFACE_STYLE_USAGE(.BOTH.,#276537);
#276537=SURFACE_SIDE_STYLE('',(#276542));
#276542=SURFACE_STYLE_FILL_AREA(#276547);
#276547=FILL_AREA_STYLE('Opaque(97,158,199)',(#276552));
#276552=FILL_AREA_STYLE_COLOUR('Opaque(97,158,199)',#276557);
#276557=COLOUR_RGB('Opaque(97,158,199)',0.380392156862745,0.619607843137255,
0.780392156862745);
ENDSEC;
END-ISO-10303-21;
